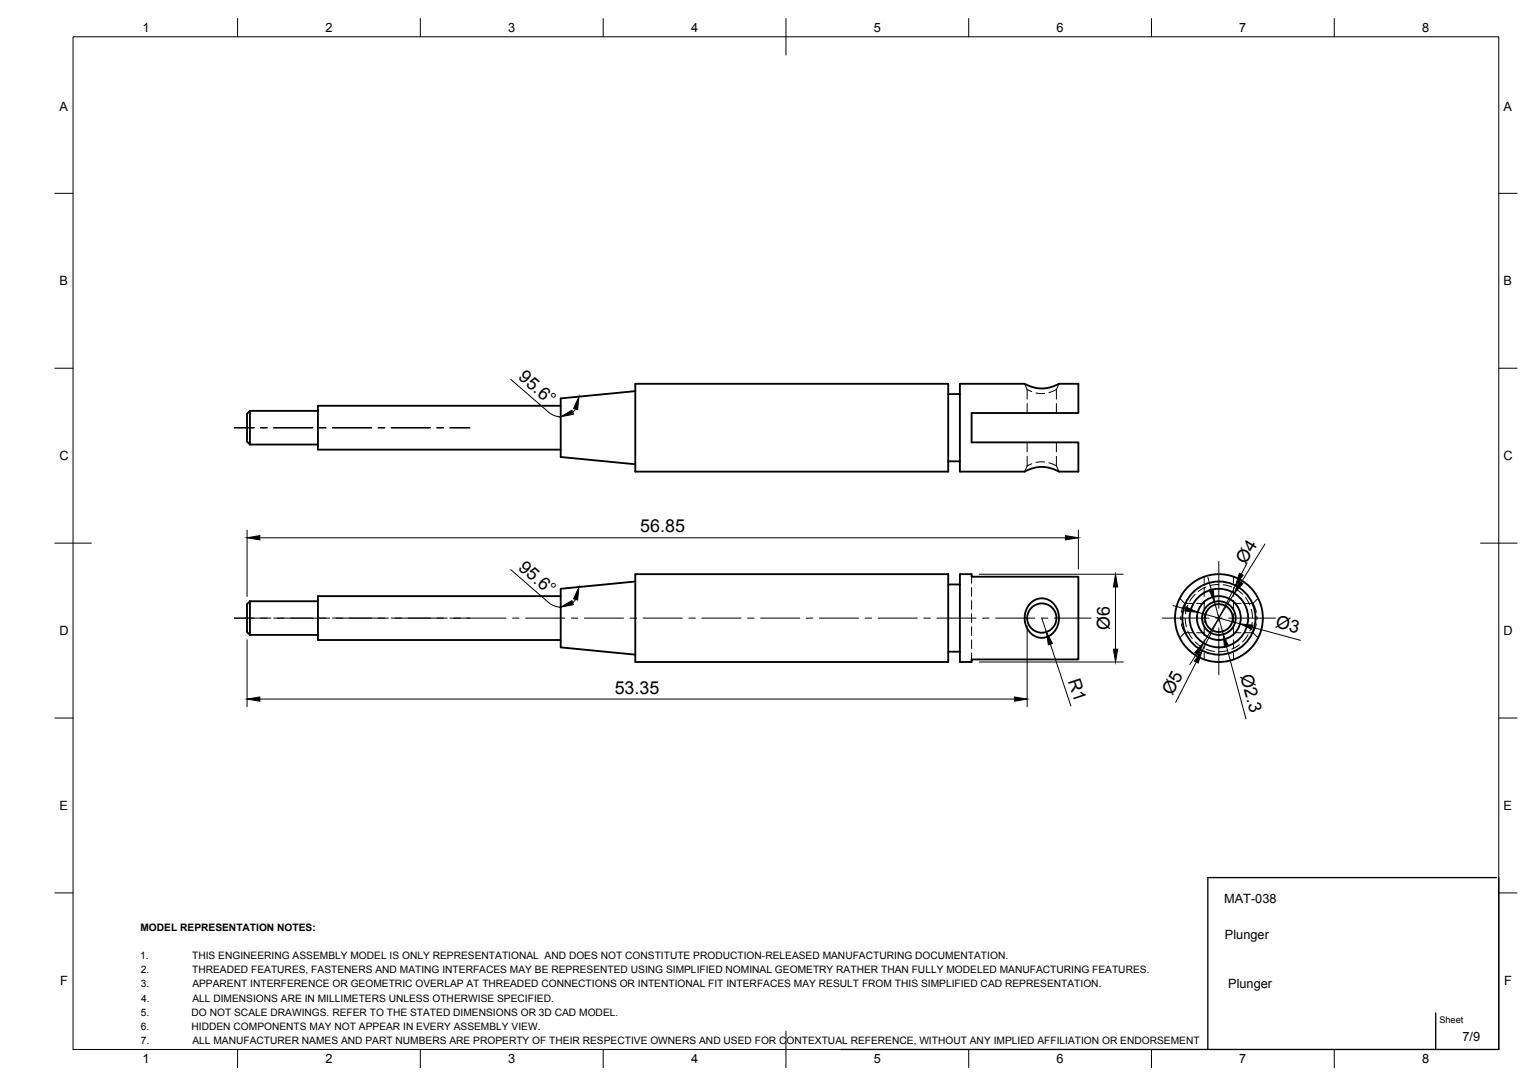
ISO-10303-21;
HEADER;
/* Generated by software containing ST-Developer
 * from STEP Tools, Inc. (www.steptools.com) 
 */

FILE_DESCRIPTION(
/* description */ ('STEP AP214'),
/* implementation_level */ '2;1');

FILE_NAME(
/* name */ 'Plunger.step',
/* time_stamp */ '2026-11-14T21:32:33-08:00',
/* author */ (''),
/* organization */ (''),
/* preprocessor_version */ 'ST-DEVELOPER v20.2',
/* originating_system */ 'Autodesk Translation Framework v15.17.0.0',
/* authorisation */ '');

FILE_SCHEMA (('AUTOMOTIVE_DESIGN { 1 0 10303 214 3 1 1 }'));
ENDSEC;

DATA;
#10=MECHANICAL_DESIGN_GEOMETRIC_PRESENTATION_REPRESENTATION('',(#181),#10551);
#135=CONICAL_SURFACE('',#3666,1.14999999999999,0.785398163397463);
#136=CONICAL_SURFACE('',#3674,1.99999999999999,0.0977269073587189);
#138=B_SPLINE_CURVE_WITH_KNOTS('',3,(#6086,#6087,#6088,#6089,#6090,#6091,
#6092,#6093,#6094,#6095,#6096,#6097,#6098,#6099,#6100,#6101,#6102,#6103,
#6104,#6105,#6106,#6107),.UNSPECIFIED.,.F.,.F.,(4,2,2,2,2,2,2,2,2,2,4),
(-0.398476386723121,-0.363413449903791,-0.328945780906488,-0.279734113540581,
-0.238759142767186,-0.202537073889496,-0.166278974820396,-0.125546922866738,
-0.0748109574930432,-0.0377065280884949,0.),.UNSPECIFIED.);
#139=B_SPLINE_CURVE_WITH_KNOTS('',3,(#6111,#6112,#6113,#6114),
 .UNSPECIFIED.,.F.,.F.,(4,4),(-0.320868204557424,-0.320859930375376),
 .UNSPECIFIED.);
#140=B_SPLINE_CURVE_WITH_KNOTS('',3,(#6116,#6117,#6118,#6119,#6120,#6121,
#6122,#6123,#6124,#6125,#6126,#6127,#6128,#6129,#6130,#6131,#6132,#6133,
#6134,#6135,#6136,#6137,#6138,#6139),.UNSPECIFIED.,.F.,.F.,(4,2,2,2,2,2,
2,2,2,2,2,4),(-0.320859930375376,-0.303821997926792,-0.286725131861031,
-0.252375001979002,-0.231369369238555,-0.194211321091721,-0.160393271457449,
-0.126524952102273,-0.0894197007003378,-0.0475320396288663,-0.0237192939459634,
-1.00000035202497E-6),.UNSPECIFIED.);
#141=B_SPLINE_CURVE_WITH_KNOTS('',3,(#6635,#6636,#6637,#6638,#6639,#6640,
#6641,#6642,#6643,#6644,#6645,#6646,#6647,#6648,#6649,#6650,#6651,#6652,
#6653,#6654,#6655,#6656),.UNSPECIFIED.,.F.,.F.,(4,2,2,2,2,2,2,2,2,2,4),
(-0.398476386717938,-0.363413449898109,-0.328945780900276,-0.279734113534564,
-0.238759142762232,-0.202537073885482,-0.166278974817291,-0.125546922864936,
-0.074810957492591,-0.0377065280884339,0.),.UNSPECIFIED.);
#142=B_SPLINE_CURVE_WITH_KNOTS('',3,(#6660,#6661,#6662,#6663),
 .UNSPECIFIED.,.F.,.F.,(4,4),(-0.320868204532271,-0.320859930350223),
 .UNSPECIFIED.);
#143=B_SPLINE_CURVE_WITH_KNOTS('',3,(#6665,#6666,#6667,#6668,#6669,#6670,
#6671,#6672,#6673,#6674,#6675,#6676,#6677,#6678,#6679,#6680,#6681,#6682,
#6683,#6684,#6685,#6686,#6687,#6688),.UNSPECIFIED.,.F.,.F.,(4,2,2,2,2,2,
2,2,2,2,2,4),(-0.320859930350223,-0.303821997902903,-0.286725131838533,
-0.252375001959359,-0.23136936922067,-0.194211321076927,-0.160393271445428,
-0.126524952093029,-0.0894197006941437,-0.0475320396261598,-0.0237192939451105,
-1.00000035191394E-6),.UNSPECIFIED.);
#144=B_SPLINE_CURVE_WITH_KNOTS('',3,(#6712,#6713,#6714,#6715,#6716,#6717,
#6718,#6719,#6720,#6721,#6722,#6723,#6724,#6725,#6726,#6727,#6728,#6729,
#6730,#6731,#6732,#6733),.UNSPECIFIED.,.F.,.F.,(4,2,2,2,2,2,2,2,2,2,4),
(-0.420674421775538,-0.382950410823496,-0.345914295714904,-0.296541537335382,
-0.257099730998724,-0.212666956872446,-0.167430581836075,-0.126839008921964,
-0.0765690827106126,-0.0387810619783508,0.),.UNSPECIFIED.);
#145=B_SPLINE_CURVE_WITH_KNOTS('',3,(#6734,#6735,#6736,#6737,#6738,#6739,
#6740,#6741,#6742,#6743,#6744,#6745,#6746,#6747,#6748,#6749,#6750,#6751,
#6752,#6753,#6754,#6755),.UNSPECIFIED.,.F.,.F.,(4,2,2,2,2,2,2,2,2,2,4),
(-0.420674421739622,-0.382950410793912,-0.345914295692047,-0.296541537321962,
-0.257099730993021,-0.212666956872502,-0.1674305818364,-0.126839008922401,
-0.0765690827112369,-0.0387810619787167,0.),.UNSPECIFIED.);
#146=B_SPLINE_CURVE_WITH_KNOTS('',3,(#6760,#6761,#6762,#6763,#6764,#6765,
#6766,#6767,#6768,#6769,#6770,#6771,#6772,#6773,#6774,#6775,#6776,#6777,
#6778,#6779,#6780,#6781),.UNSPECIFIED.,.F.,.F.,(4,2,2,2,2,2,2,2,2,2,4),
(1.00000051704647E-6,0.0346979268821443,0.0692680598480025,0.109244972085431,
0.144041383182867,0.160697846212527,0.177234449156828,0.212032576255554,
0.252099494752921,0.286510766916454,0.320844032281287),.UNSPECIFIED.);
#147=B_SPLINE_CURVE_WITH_KNOTS('',3,(#6786,#6787,#6788,#6789,#6790,#6791,
#6792,#6793,#6794,#6795,#6796,#6797,#6798,#6799,#6800,#6801,#6802,#6803,
#6804,#6805,#6806,#6807),.UNSPECIFIED.,.F.,.F.,(4,2,2,2,2,2,2,2,2,2,4),
(1.00000051707666E-6,0.0346979268820894,0.0692680598476906,0.109244972084642,
0.14404138318175,0.160697846211195,0.17723444915527,0.212032576253597,0.252099494750475,
0.286510766913486,0.3208440322786),.UNSPECIFIED.);
#155=B_SPLINE_SURFACE_WITH_KNOTS('',1,3,((#5592,#5593,#5594,#5595,#5596,
#5597,#5598,#5599,#5600,#5601,#5602,#5603,#5604,#5605,#5606,#5607,#5608,
#5609,#5610,#5611,#5612,#5613,#5614,#5615,#5616,#5617,#5618,#5619,#5620,
#5621,#5622,#5623,#5624,#5625,#5626,#5627,#5628,#5629,#5630,#5631,#5632,
#5633,#5634,#5635,#5636,#5637,#5638,#5639,#5640,#5641,#5642,#5643,#5644,
#5645,#5646,#5647,#5648,#5649,#5650,#5651,#5652,#5653,#5654,#5655,#5656,
#5657,#5658,#5659,#5660,#5661,#5662,#5663,#5664,#5665,#5666,#5667,#5668,
#5669,#5670,#5671,#5672,#5673,#5674,#5675,#5676,#5677,#5678,#5679,#5680,
#5681,#5682,#5683,#5684,#5685,#5686,#5687,#5688,#5689,#5690,#5691,#5692,
#5693,#5694,#5695,#5696,#5697,#5698,#5699,#5700,#5701,#5702,#5703,#5704,
#5705,#5706,#5707,#5708,#5709,#5710,#5711,#5712,#5713,#5714,#5715,#5716,
#5717,#5718,#5719,#5720,#5721,#5722,#5723,#5724,#5725,#5726,#5727,#5728,
#5729,#5730,#5731,#5732,#5733,#5734,#5735,#5736,#5737,#5738,#5739,#5740,
#5741,#5742,#5743,#5744,#5745,#5746,#5747,#5748,#5749,#5750,#5751,#5752,
#5753,#5754,#5755,#5756,#5757,#5758,#5759,#5760,#5761,#5762,#5763,#5764,
#5765,#5766,#5767,#5768,#5769,#5770,#5771,#5772,#5773,#5774,#5775,#5776,
#5777,#5778,#5779,#5780,#5781,#5782,#5783,#5784,#5785,#5786,#5787,#5788,
#5789,#5790,#5791,#5792,#5793,#5794,#5795,#5796,#5797,#5798,#5799,#5800,
#5801,#5802,#5803,#5804,#5805,#5806,#5807,#5808,#5809,#5810,#5811,#5812,
#5813,#5814,#5815,#5816,#5817,#5818,#5819,#5820,#5821,#5822,#5823,#5824,
#5825,#5826,#5827,#5828,#5829,#5830,#5831,#5832,#5833,#5834,#5835,#5836,
#5837),(#5838,#5839,#5840,#5841,#5842,#5843,#5844,#5845,#5846,#5847,#5848,
#5849,#5850,#5851,#5852,#5853,#5854,#5855,#5856,#5857,#5858,#5859,#5860,
#5861,#5862,#5863,#5864,#5865,#5866,#5867,#5868,#5869,#5870,#5871,#5872,
#5873,#5874,#5875,#5876,#5877,#5878,#5879,#5880,#5881,#5882,#5883,#5884,
#5885,#5886,#5887,#5888,#5889,#5890,#5891,#5892,#5893,#5894,#5895,#5896,
#5897,#5898,#5899,#5900,#5901,#5902,#5903,#5904,#5905,#5906,#5907,#5908,
#5909,#5910,#5911,#5912,#5913,#5914,#5915,#5916,#5917,#5918,#5919,#5920,
#5921,#5922,#5923,#5924,#5925,#5926,#5927,#5928,#5929,#5930,#5931,#5932,
#5933,#5934,#5935,#5936,#5937,#5938,#5939,#5940,#5941,#5942,#5943,#5944,
#5945,#5946,#5947,#5948,#5949,#5950,#5951,#5952,#5953,#5954,#5955,#5956,
#5957,#5958,#5959,#5960,#5961,#5962,#5963,#5964,#5965,#5966,#5967,#5968,
#5969,#5970,#5971,#5972,#5973,#5974,#5975,#5976,#5977,#5978,#5979,#5980,
#5981,#5982,#5983,#5984,#5985,#5986,#5987,#5988,#5989,#5990,#5991,#5992,
#5993,#5994,#5995,#5996,#5997,#5998,#5999,#6000,#6001,#6002,#6003,#6004,
#6005,#6006,#6007,#6008,#6009,#6010,#6011,#6012,#6013,#6014,#6015,#6016,
#6017,#6018,#6019,#6020,#6021,#6022,#6023,#6024,#6025,#6026,#6027,#6028,
#6029,#6030,#6031,#6032,#6033,#6034,#6035,#6036,#6037,#6038,#6039,#6040,
#6041,#6042,#6043,#6044,#6045,#6046,#6047,#6048,#6049,#6050,#6051,#6052,
#6053,#6054,#6055,#6056,#6057,#6058,#6059,#6060,#6061,#6062,#6063,#6064,
#6065,#6066,#6067,#6068,#6069,#6070,#6071,#6072,#6073,#6074,#6075,#6076,
#6077,#6078,#6079,#6080,#6081,#6082,#6083)),.UNSPECIFIED.,.F.,.T.,.F.,(2,
2),(4,2,2,2,2,2,2,2,2,2,2,2,2,2,2,2,2,2,2,2,2,2,2,2,2,2,2,2,2,2,2,2,2,2,
2,2,2,2,2,2,2,2,2,2,2,2,2,2,2,2,2,2,2,2,2,2,2,2,2,2,2,2,2,2,2,2,2,2,2,2,
2,2,2,2,2,2,2,2,2,2,2,2,2,2,2,2,2,2,2,2,2,2,2,2,2,2,2,2,2,2,2,2,2,2,2,2,
2,2,2,2,2,2,2,2,2,2,2,2,2,2,2,2,4),(-1.00016962386399E-6,1.),(0.000438425814883596,
0.00049639971234602,0.000554373609808444,0.000670321404733293,0.000728295302195718,
0.00075728225092693,0.000786269199658142,0.000844243097120567,0.000902216994582991,
0.00101816478950784,0.00107613868697026,0.00113411258443269,0.00119208648189511,
0.00125006037935754,0.00136600817428239,0.00142398207174481,0.00148195596920724,
0.00153992986666966,0.00159790376413208,0.00165587766159451,0.00171385155905693,
0.00182979935398178,0.00188777325144421,0.00191676020017542,0.00194574714890663,
0.00200372104636906,0.00206169494383148,0.00217764273875633,0.00223561663621875,
0.00229359053368118,0.0023515644311436,0.00240953832860603,0.00246751222606845,
0.00252548612353088,0.00264143391845572,0.00267042086718694,0.00269940781591815,
0.00275738171338057,0.002815355610843,0.00287332950830542,0.00293130340576785,
0.00298927730323027,0.0030472512006927,0.00310522509815512,0.00316319899561754,
0.00322117289307997,0.00333712068800482,0.00339509458546724,0.00342408153419845,
0.00345306848292967,0.00351104238039209,0.00356901627785452,0.00368496407277936,
0.00380091186770421,0.00385888576516664,0.00391685966262906,0.00397483356009149,
0.00403280745755391,0.00414875525247876,0.00420672914994119,0.00426470304740361,
0.00432267694486603,0.00438065084232846,0.00443862473979088,0.00449659863725331,
0.00461254643217816,0.00467052032964058,0.00469950727837179,0.00472849422710301,
0.00478646812456543,0.00484444202202785,0.0049603898169527,0.00501836371441513,
0.00507633761187755,0.00510532456060876,0.00513431150933998,0.0051922854068024,
0.00530823320172725,0.00536620709918968,0.0054241809966521,0.00548215489411452,
0.00551114184284574,0.00554012879157695,0.0056560765865018,0.00577202438142665,
0.00582999827888907,0.00588797217635149,0.00591695912508271,0.00594594607381392,
0.00600391997127634,0.00611986776620119,0.00617784166366362,0.00623581556112604,
0.00626480250985725,0.00629378945858847,0.00635176335605089,0.00640973725351331,
0.00646771115097574,0.00658365894590059,0.0066126458946318,0.00664163284336301,
0.00669960674082544,0.00675758063828786,0.00681555453575028,0.00687352843321271,
0.00693150233067513,0.00698947622813756,0.00701846317686877,0.00704745012559998,
0.00716339792052483,0.00727934571544968,0.0073373196129121,0.00739529351037453,
0.00742428045910574,0.00745326740783695,0.00751124130529938,0.0075692152027618,
0.00762718910022423,0.00768516299768665,0.00774313689514908,0.0078011107926115,
0.00783009774134271,0.00785908469007393),.UNSPECIFIED.);
#156=B_SPLINE_SURFACE_WITH_KNOTS('',1,3,((#6141,#6142,#6143,#6144,#6145,
#6146,#6147,#6148,#6149,#6150,#6151,#6152,#6153,#6154,#6155,#6156,#6157,
#6158,#6159,#6160,#6161,#6162,#6163,#6164,#6165,#6166,#6167,#6168,#6169,
#6170,#6171,#6172,#6173,#6174,#6175,#6176,#6177,#6178,#6179,#6180,#6181,
#6182,#6183,#6184,#6185,#6186,#6187,#6188,#6189,#6190,#6191,#6192,#6193,
#6194,#6195,#6196,#6197,#6198,#6199,#6200,#6201,#6202,#6203,#6204,#6205,
#6206,#6207,#6208,#6209,#6210,#6211,#6212,#6213,#6214,#6215,#6216,#6217,
#6218,#6219,#6220,#6221,#6222,#6223,#6224,#6225,#6226,#6227,#6228,#6229,
#6230,#6231,#6232,#6233,#6234,#6235,#6236,#6237,#6238,#6239,#6240,#6241,
#6242,#6243,#6244,#6245,#6246,#6247,#6248,#6249,#6250,#6251,#6252,#6253,
#6254,#6255,#6256,#6257,#6258,#6259,#6260,#6261,#6262,#6263,#6264,#6265,
#6266,#6267,#6268,#6269,#6270,#6271,#6272,#6273,#6274,#6275,#6276,#6277,
#6278,#6279,#6280,#6281,#6282,#6283,#6284,#6285,#6286,#6287,#6288,#6289,
#6290,#6291,#6292,#6293,#6294,#6295,#6296,#6297,#6298,#6299,#6300,#6301,
#6302,#6303,#6304,#6305,#6306,#6307,#6308,#6309,#6310,#6311,#6312,#6313,
#6314,#6315,#6316,#6317,#6318,#6319,#6320,#6321,#6322,#6323,#6324,#6325,
#6326,#6327,#6328,#6329,#6330,#6331,#6332,#6333,#6334,#6335,#6336,#6337,
#6338,#6339,#6340,#6341,#6342,#6343,#6344,#6345,#6346,#6347,#6348,#6349,
#6350,#6351,#6352,#6353,#6354,#6355,#6356,#6357,#6358,#6359,#6360,#6361,
#6362,#6363,#6364,#6365,#6366,#6367,#6368,#6369,#6370,#6371,#6372,#6373,
#6374,#6375,#6376,#6377,#6378,#6379,#6380,#6381,#6382,#6383,#6384,#6385,
#6386),(#6387,#6388,#6389,#6390,#6391,#6392,#6393,#6394,#6395,#6396,#6397,
#6398,#6399,#6400,#6401,#6402,#6403,#6404,#6405,#6406,#6407,#6408,#6409,
#6410,#6411,#6412,#6413,#6414,#6415,#6416,#6417,#6418,#6419,#6420,#6421,
#6422,#6423,#6424,#6425,#6426,#6427,#6428,#6429,#6430,#6431,#6432,#6433,
#6434,#6435,#6436,#6437,#6438,#6439,#6440,#6441,#6442,#6443,#6444,#6445,
#6446,#6447,#6448,#6449,#6450,#6451,#6452,#6453,#6454,#6455,#6456,#6457,
#6458,#6459,#6460,#6461,#6462,#6463,#6464,#6465,#6466,#6467,#6468,#6469,
#6470,#6471,#6472,#6473,#6474,#6475,#6476,#6477,#6478,#6479,#6480,#6481,
#6482,#6483,#6484,#6485,#6486,#6487,#6488,#6489,#6490,#6491,#6492,#6493,
#6494,#6495,#6496,#6497,#6498,#6499,#6500,#6501,#6502,#6503,#6504,#6505,
#6506,#6507,#6508,#6509,#6510,#6511,#6512,#6513,#6514,#6515,#6516,#6517,
#6518,#6519,#6520,#6521,#6522,#6523,#6524,#6525,#6526,#6527,#6528,#6529,
#6530,#6531,#6532,#6533,#6534,#6535,#6536,#6537,#6538,#6539,#6540,#6541,
#6542,#6543,#6544,#6545,#6546,#6547,#6548,#6549,#6550,#6551,#6552,#6553,
#6554,#6555,#6556,#6557,#6558,#6559,#6560,#6561,#6562,#6563,#6564,#6565,
#6566,#6567,#6568,#6569,#6570,#6571,#6572,#6573,#6574,#6575,#6576,#6577,
#6578,#6579,#6580,#6581,#6582,#6583,#6584,#6585,#6586,#6587,#6588,#6589,
#6590,#6591,#6592,#6593,#6594,#6595,#6596,#6597,#6598,#6599,#6600,#6601,
#6602,#6603,#6604,#6605,#6606,#6607,#6608,#6609,#6610,#6611,#6612,#6613,
#6614,#6615,#6616,#6617,#6618,#6619,#6620,#6621,#6622,#6623,#6624,#6625,
#6626,#6627,#6628,#6629,#6630,#6631,#6632)),.UNSPECIFIED.,.F.,.T.,.F.,(2,
2),(4,2,2,2,2,2,2,2,2,2,2,2,2,2,2,2,2,2,2,2,2,2,2,2,2,2,2,2,2,2,2,2,2,2,
2,2,2,2,2,2,2,2,2,2,2,2,2,2,2,2,2,2,2,2,2,2,2,2,2,2,2,2,2,2,2,2,2,2,2,2,
2,2,2,2,2,2,2,2,2,2,2,2,2,2,2,2,2,2,2,2,2,2,2,2,2,2,2,2,2,2,2,2,2,2,2,2,
2,2,2,2,2,2,2,2,2,2,2,2,2,2,2,2,4),(-1.00016962714665E-6,1.),(0.000438425814883592,
0.000496399712346016,0.000554373609808441,0.000670321404733289,0.000728295302195713,
0.000757282250926925,0.000786269199658137,0.000844243097120562,0.000902216994582986,
0.00101816478950783,0.00107613868697026,0.00113411258443268,0.00119208648189511,
0.00125006037935753,0.00136600817428238,0.0014239820717448,0.00148195596920723,
0.00153992986666965,0.00159790376413208,0.0016558776615945,0.00171385155905693,
0.00182979935398177,0.0018877732514442,0.00191676020017541,0.00194574714890662,
0.00200372104636905,0.00206169494383147,0.00217764273875632,0.00223561663621874,
0.00229359053368117,0.00235156443114359,0.00240953832860602,0.00246751222606844,
0.00252548612353086,0.00264143391845571,0.00267042086718692,0.00269940781591814,
0.00275738171338056,0.00281535561084298,0.00287332950830541,0.00293130340576783,
0.00298927730323026,0.00304725120069268,0.00310522509815511,0.00316319899561753,
0.00322117289307996,0.0033371206880048,0.00339509458546723,0.00342408153419844,
0.00345306848292965,0.00351104238039208,0.0035690162778545,0.00368496407277935,
0.0038009118677042,0.00385888576516662,0.00391685966262905,0.00397483356009147,
0.00403280745755389,0.00414875525247874,0.00420672914994117,0.00426470304740359,
0.00432267694486602,0.00438065084232844,0.00443862473979086,0.00449659863725329,
0.00461254643217814,0.00467052032964056,0.00469950727837177,0.00472849422710298,
0.00478646812456541,0.00484444202202783,0.00496038981695268,0.00501836371441511,
0.00507633761187753,0.00510532456060874,0.00513431150933995,0.00519228540680238,
0.00530823320172723,0.00536620709918965,0.00542418099665208,0.0054821548941145,
0.00551114184284571,0.00554012879157692,0.00565607658650177,0.00577202438142662,
0.00582999827888904,0.00588797217635147,0.00591695912508268,0.00594594607381389,
0.00600391997127632,0.00611986776620117,0.00617784166366359,0.00623581556112602,
0.00626480250985723,0.00629378945858844,0.00635176335605086,0.00640973725351329,
0.00646771115097571,0.00658365894590056,0.00661264589463177,0.00664163284336298,
0.00669960674082541,0.00675758063828783,0.00681555453575026,0.00687352843321268,
0.00693150233067511,0.00698947622813753,0.00701846317686874,0.00704745012559995,
0.0071633979205248,0.00727934571544965,0.00733731961291207,0.0073952935103745,
0.00742428045910571,0.00745326740783692,0.00751124130529935,0.00756921520276177,
0.0076271891002242,0.00768516299768662,0.00774313689514904,0.00780111079261147,
0.00783009774134268,0.00785908469007389),.UNSPECIFIED.);
#157=B_SPLINE_SURFACE_WITH_KNOTS('',1,3,((#6848,#6849,#6850,#6851,#6852,
#6853,#6854,#6855,#6856,#6857,#6858,#6859,#6860,#6861,#6862,#6863,#6864,
#6865,#6866,#6867,#6868,#6869,#6870,#6871,#6872,#6873,#6874,#6875,#6876,
#6877,#6878,#6879,#6880,#6881,#6882,#6883,#6884,#6885,#6886,#6887,#6888,
#6889,#6890,#6891,#6892,#6893,#6894,#6895,#6896,#6897,#6898,#6899,#6900,
#6901,#6902,#6903,#6904,#6905,#6906,#6907,#6908,#6909,#6910,#6911,#6912,
#6913,#6914,#6915,#6916,#6917,#6918,#6919,#6920,#6921,#6922,#6923,#6924,
#6925,#6926,#6927,#6928,#6929,#6930,#6931,#6932,#6933,#6934,#6935,#6936,
#6937,#6938,#6939,#6940,#6941,#6942,#6943,#6944,#6945,#6946,#6947,#6948,
#6949,#6950,#6951,#6952,#6953,#6954,#6955,#6956,#6957,#6958,#6959,#6960,
#6961,#6962,#6963,#6964,#6965,#6966,#6967,#6968,#6969,#6970,#6971,#6972,
#6973,#6974,#6975,#6976,#6977,#6978,#6979,#6980,#6981,#6982,#6983,#6984,
#6985,#6986,#6987,#6988,#6989,#6990,#6991,#6992,#6993,#6994,#6995,#6996,
#6997,#6998,#6999,#7000,#7001,#7002,#7003,#7004,#7005,#7006,#7007,#7008,
#7009,#7010,#7011,#7012,#7013,#7014,#7015,#7016,#7017,#7018,#7019,#7020,
#7021,#7022,#7023,#7024,#7025,#7026,#7027,#7028,#7029,#7030,#7031,#7032,
#7033,#7034,#7035,#7036,#7037,#7038,#7039,#7040,#7041,#7042,#7043,#7044,
#7045,#7046,#7047,#7048,#7049,#7050,#7051,#7052,#7053,#7054,#7055,#7056,
#7057,#7058,#7059,#7060,#7061,#7062,#7063,#7064,#7065,#7066,#7067,#7068,
#7069,#7070,#7071,#7072,#7073,#7074,#7075,#7076,#7077,#7078,#7079,#7080,
#7081,#7082,#7083,#7084,#7085,#7086,#7087,#7088,#7089,#7090,#7091,#7092,
#7093),(#7094,#7095,#7096,#7097,#7098,#7099,#7100,#7101,#7102,#7103,#7104,
#7105,#7106,#7107,#7108,#7109,#7110,#7111,#7112,#7113,#7114,#7115,#7116,
#7117,#7118,#7119,#7120,#7121,#7122,#7123,#7124,#7125,#7126,#7127,#7128,
#7129,#7130,#7131,#7132,#7133,#7134,#7135,#7136,#7137,#7138,#7139,#7140,
#7141,#7142,#7143,#7144,#7145,#7146,#7147,#7148,#7149,#7150,#7151,#7152,
#7153,#7154,#7155,#7156,#7157,#7158,#7159,#7160,#7161,#7162,#7163,#7164,
#7165,#7166,#7167,#7168,#7169,#7170,#7171,#7172,#7173,#7174,#7175,#7176,
#7177,#7178,#7179,#7180,#7181,#7182,#7183,#7184,#7185,#7186,#7187,#7188,
#7189,#7190,#7191,#7192,#7193,#7194,#7195,#7196,#7197,#7198,#7199,#7200,
#7201,#7202,#7203,#7204,#7205,#7206,#7207,#7208,#7209,#7210,#7211,#7212,
#7213,#7214,#7215,#7216,#7217,#7218,#7219,#7220,#7221,#7222,#7223,#7224,
#7225,#7226,#7227,#7228,#7229,#7230,#7231,#7232,#7233,#7234,#7235,#7236,
#7237,#7238,#7239,#7240,#7241,#7242,#7243,#7244,#7245,#7246,#7247,#7248,
#7249,#7250,#7251,#7252,#7253,#7254,#7255,#7256,#7257,#7258,#7259,#7260,
#7261,#7262,#7263,#7264,#7265,#7266,#7267,#7268,#7269,#7270,#7271,#7272,
#7273,#7274,#7275,#7276,#7277,#7278,#7279,#7280,#7281,#7282,#7283,#7284,
#7285,#7286,#7287,#7288,#7289,#7290,#7291,#7292,#7293,#7294,#7295,#7296,
#7297,#7298,#7299,#7300,#7301,#7302,#7303,#7304,#7305,#7306,#7307,#7308,
#7309,#7310,#7311,#7312,#7313,#7314,#7315,#7316,#7317,#7318,#7319,#7320,
#7321,#7322,#7323,#7324,#7325,#7326,#7327,#7328,#7329,#7330,#7331,#7332,
#7333,#7334,#7335,#7336,#7337,#7338,#7339)),.UNSPECIFIED.,.F.,.T.,.F.,(2,
2),(4,2,2,2,2,2,2,2,2,2,2,2,2,2,2,2,2,2,2,2,2,2,2,2,2,2,2,2,2,2,2,2,2,2,
2,2,2,2,2,2,2,2,2,2,2,2,2,2,2,2,2,2,2,2,2,2,2,2,2,2,2,2,2,2,2,2,2,2,2,2,
2,2,2,2,2,2,2,2,2,2,2,2,2,2,2,2,2,2,2,2,2,2,2,2,2,2,2,2,2,2,2,2,2,2,2,2,
2,2,2,2,2,2,2,2,2,2,2,2,2,2,2,2,4),(-3.16760819181413E-6,1.00000897992091),
(0.000438425814883592,0.000496399712346016,0.000554373609808441,0.000670321404733289,
0.000728295302195713,0.000757282250926925,0.000786269199658137,0.000844243097120562,
0.000902216994582986,0.00101816478950783,0.00107613868697026,0.00113411258443268,
0.00119208648189511,0.00125006037935753,0.00136600817428238,0.0014239820717448,
0.00148195596920723,0.00153992986666965,0.00159790376413208,0.0016558776615945,
0.00171385155905693,0.00182979935398177,0.0018877732514442,0.00191676020017541,
0.00194574714890662,0.00200372104636905,0.00206169494383147,0.00217764273875632,
0.00223561663621874,0.00229359053368117,0.00235156443114359,0.00240953832860602,
0.00246751222606844,0.00252548612353086,0.00264143391845571,0.00267042086718692,
0.00269940781591814,0.00275738171338056,0.00281535561084298,0.00287332950830541,
0.00293130340576783,0.00298927730323026,0.00304725120069268,0.00310522509815511,
0.00316319899561753,0.00322117289307996,0.0033371206880048,0.00339509458546723,
0.00342408153419844,0.00345306848292965,0.00351104238039208,0.0035690162778545,
0.00368496407277935,0.0038009118677042,0.00385888576516662,0.00391685966262905,
0.00397483356009147,0.00403280745755389,0.00414875525247874,0.00420672914994117,
0.00426470304740359,0.00432267694486602,0.00438065084232844,0.00443862473979086,
0.00449659863725329,0.00461254643217814,0.00467052032964056,0.00469950727837177,
0.00472849422710298,0.00478646812456541,0.00484444202202783,0.00496038981695268,
0.00501836371441511,0.00507633761187753,0.00510532456060874,0.00513431150933995,
0.00519228540680238,0.00530823320172723,0.00536620709918965,0.00542418099665208,
0.0054821548941145,0.00551114184284571,0.00554012879157692,0.00565607658650177,
0.00577202438142662,0.00582999827888904,0.00588797217635147,0.00591695912508268,
0.00594594607381389,0.00600391997127632,0.00611986776620117,0.00617784166366359,
0.00623581556112602,0.00626480250985723,0.00629378945858844,0.00635176335605086,
0.00640973725351329,0.00646771115097571,0.00658365894590056,0.00661264589463177,
0.00664163284336298,0.00669960674082541,0.00675758063828783,0.00681555453575026,
0.00687352843321268,0.00693150233067511,0.00698947622813753,0.00701846317686874,
0.00704745012559995,0.0071633979205248,0.00727934571544965,0.00733731961291207,
0.0073952935103745,0.00742428045910571,0.00745326740783692,0.00751124130529935,
0.00756921520276177,0.0076271891002242,0.00768516299768662,0.00774313689514904,
0.00780111079261147,0.00783009774134268,0.00785908469007389),
 .UNSPECIFIED.);
#158=B_SPLINE_SURFACE_WITH_KNOTS('',1,3,((#7340,#7341,#7342,#7343,#7344,
#7345,#7346,#7347,#7348,#7349,#7350,#7351,#7352,#7353,#7354,#7355,#7356,
#7357,#7358,#7359,#7360,#7361,#7362,#7363,#7364,#7365,#7366,#7367,#7368,
#7369,#7370,#7371,#7372,#7373,#7374,#7375,#7376,#7377,#7378,#7379,#7380,
#7381,#7382,#7383,#7384,#7385,#7386,#7387,#7388,#7389,#7390,#7391,#7392,
#7393,#7394,#7395,#7396,#7397,#7398,#7399,#7400,#7401,#7402,#7403,#7404,
#7405,#7406,#7407,#7408,#7409,#7410,#7411,#7412,#7413,#7414,#7415,#7416,
#7417,#7418,#7419,#7420,#7421,#7422,#7423,#7424,#7425,#7426,#7427,#7428,
#7429,#7430,#7431,#7432,#7433,#7434,#7435,#7436,#7437,#7438,#7439,#7440,
#7441,#7442,#7443,#7444,#7445,#7446,#7447,#7448,#7449,#7450,#7451,#7452,
#7453,#7454,#7455,#7456,#7457,#7458,#7459,#7460,#7461,#7462,#7463,#7464,
#7465,#7466,#7467,#7468,#7469,#7470,#7471,#7472,#7473,#7474,#7475,#7476,
#7477,#7478,#7479,#7480,#7481,#7482,#7483,#7484,#7485,#7486,#7487,#7488,
#7489,#7490,#7491,#7492,#7493,#7494,#7495,#7496,#7497,#7498,#7499,#7500,
#7501,#7502,#7503,#7504,#7505,#7506,#7507,#7508,#7509,#7510,#7511,#7512,
#7513,#7514,#7515,#7516,#7517,#7518,#7519,#7520,#7521,#7522,#7523,#7524,
#7525,#7526,#7527,#7528,#7529,#7530,#7531,#7532,#7533,#7534,#7535,#7536,
#7537,#7538,#7539,#7540,#7541,#7542,#7543,#7544,#7545,#7546,#7547,#7548,
#7549,#7550,#7551,#7552,#7553,#7554,#7555,#7556,#7557,#7558,#7559,#7560,
#7561,#7562,#7563,#7564,#7565,#7566,#7567,#7568,#7569,#7570,#7571,#7572,
#7573,#7574,#7575,#7576,#7577,#7578,#7579,#7580,#7581,#7582,#7583,#7584,
#7585),(#7586,#7587,#7588,#7589,#7590,#7591,#7592,#7593,#7594,#7595,#7596,
#7597,#7598,#7599,#7600,#7601,#7602,#7603,#7604,#7605,#7606,#7607,#7608,
#7609,#7610,#7611,#7612,#7613,#7614,#7615,#7616,#7617,#7618,#7619,#7620,
#7621,#7622,#7623,#7624,#7625,#7626,#7627,#7628,#7629,#7630,#7631,#7632,
#7633,#7634,#7635,#7636,#7637,#7638,#7639,#7640,#7641,#7642,#7643,#7644,
#7645,#7646,#7647,#7648,#7649,#7650,#7651,#7652,#7653,#7654,#7655,#7656,
#7657,#7658,#7659,#7660,#7661,#7662,#7663,#7664,#7665,#7666,#7667,#7668,
#7669,#7670,#7671,#7672,#7673,#7674,#7675,#7676,#7677,#7678,#7679,#7680,
#7681,#7682,#7683,#7684,#7685,#7686,#7687,#7688,#7689,#7690,#7691,#7692,
#7693,#7694,#7695,#7696,#7697,#7698,#7699,#7700,#7701,#7702,#7703,#7704,
#7705,#7706,#7707,#7708,#7709,#7710,#7711,#7712,#7713,#7714,#7715,#7716,
#7717,#7718,#7719,#7720,#7721,#7722,#7723,#7724,#7725,#7726,#7727,#7728,
#7729,#7730,#7731,#7732,#7733,#7734,#7735,#7736,#7737,#7738,#7739,#7740,
#7741,#7742,#7743,#7744,#7745,#7746,#7747,#7748,#7749,#7750,#7751,#7752,
#7753,#7754,#7755,#7756,#7757,#7758,#7759,#7760,#7761,#7762,#7763,#7764,
#7765,#7766,#7767,#7768,#7769,#7770,#7771,#7772,#7773,#7774,#7775,#7776,
#7777,#7778,#7779,#7780,#7781,#7782,#7783,#7784,#7785,#7786,#7787,#7788,
#7789,#7790,#7791,#7792,#7793,#7794,#7795,#7796,#7797,#7798,#7799,#7800,
#7801,#7802,#7803,#7804,#7805,#7806,#7807,#7808,#7809,#7810,#7811,#7812,
#7813,#7814,#7815,#7816,#7817,#7818,#7819,#7820,#7821,#7822,#7823,#7824,
#7825,#7826,#7827,#7828,#7829,#7830,#7831)),.UNSPECIFIED.,.F.,.T.,.F.,(2,
2),(4,2,2,2,2,2,2,2,2,2,2,2,2,2,2,2,2,2,2,2,2,2,2,2,2,2,2,2,2,2,2,2,2,2,
2,2,2,2,2,2,2,2,2,2,2,2,2,2,2,2,2,2,2,2,2,2,2,2,2,2,2,2,2,2,2,2,2,2,2,2,
2,2,2,2,2,2,2,2,2,2,2,2,2,2,2,2,2,2,2,2,2,2,2,2,2,2,2,2,2,2,2,2,2,2,2,2,
2,2,2,2,2,2,2,2,2,2,2,2,2,2,2,2,4),(-3.16760819184598E-6,1.00000897992087),
(0.000438425814883596,0.00049639971234602,0.000554373609808444,0.000670321404733293,
0.000728295302195718,0.00075728225092693,0.000786269199658142,0.000844243097120567,
0.000902216994582991,0.00101816478950784,0.00107613868697026,0.00113411258443269,
0.00119208648189511,0.00125006037935754,0.00136600817428239,0.00142398207174481,
0.00148195596920724,0.00153992986666966,0.00159790376413208,0.00165587766159451,
0.00171385155905693,0.00182979935398178,0.00188777325144421,0.00191676020017542,
0.00194574714890663,0.00200372104636906,0.00206169494383148,0.00217764273875633,
0.00223561663621875,0.00229359053368118,0.0023515644311436,0.00240953832860603,
0.00246751222606845,0.00252548612353088,0.00264143391845572,0.00267042086718694,
0.00269940781591815,0.00275738171338057,0.002815355610843,0.00287332950830542,
0.00293130340576785,0.00298927730323027,0.0030472512006927,0.00310522509815512,
0.00316319899561754,0.00322117289307997,0.00333712068800482,0.00339509458546724,
0.00342408153419845,0.00345306848292967,0.00351104238039209,0.00356901627785452,
0.00368496407277936,0.00380091186770421,0.00385888576516664,0.00391685966262906,
0.00397483356009149,0.00403280745755391,0.00414875525247876,0.00420672914994119,
0.00426470304740361,0.00432267694486603,0.00438065084232846,0.00443862473979088,
0.00449659863725331,0.00461254643217816,0.00467052032964058,0.00469950727837179,
0.00472849422710301,0.00478646812456543,0.00484444202202785,0.0049603898169527,
0.00501836371441513,0.00507633761187755,0.00510532456060876,0.00513431150933998,
0.0051922854068024,0.00530823320172725,0.00536620709918968,0.0054241809966521,
0.00548215489411452,0.00551114184284574,0.00554012879157695,0.0056560765865018,
0.00577202438142665,0.00582999827888907,0.00588797217635149,0.00591695912508271,
0.00594594607381392,0.00600391997127634,0.00611986776620119,0.00617784166366362,
0.00623581556112604,0.00626480250985725,0.00629378945858847,0.00635176335605089,
0.00640973725351331,0.00646771115097574,0.00658365894590059,0.0066126458946318,
0.00664163284336301,0.00669960674082544,0.00675758063828786,0.00681555453575028,
0.00687352843321271,0.00693150233067513,0.00698947622813756,0.00701846317686877,
0.00704745012559998,0.00716339792052483,0.00727934571544968,0.0073373196129121,
0.00739529351037453,0.00742428045910574,0.00745326740783695,0.00751124130529938,
0.0075692152027618,0.00762718910022423,0.00768516299768665,0.00774313689514908,
0.0078011107926115,0.00783009774134271,0.00785908469007393),
 .UNSPECIFIED.);
#163=SHAPE_REPRESENTATION_RELATIONSHIP('SRR','None',#10590,#172);
#172=ADVANCED_BREP_SHAPE_REPRESENTATION('',(#191),#10546);
#181=STYLED_ITEM('',(#10643),#191);
#191=MANIFOLD_SOLID_BREP('Body1',#3430);
#212=FACE_BOUND('',#600,.T.);
#213=FACE_BOUND('',#601,.T.);
#214=FACE_BOUND('',#611,.T.);
#215=FACE_BOUND('',#613,.T.);
#216=FACE_BOUND('',#615,.T.);
#217=FACE_BOUND('',#618,.T.);
#218=FACE_BOUND('',#620,.T.);
#219=FACE_BOUND('',#625,.T.);
#220=FACE_BOUND('',#628,.T.);
#271=PLANE('',#3680);
#272=PLANE('',#3681);
#273=PLANE('',#3682);
#274=PLANE('',#3683);
#275=PLANE('',#3684);
#276=PLANE('',#3685);
#277=PLANE('',#3686);
#278=PLANE('',#3687);
#279=PLANE('',#3688);
#280=PLANE('',#3689);
#281=PLANE('',#3690);
#362=FACE_OUTER_BOUND('',#597,.T.);
#363=FACE_OUTER_BOUND('',#598,.T.);
#364=FACE_OUTER_BOUND('',#599,.T.);
#365=FACE_OUTER_BOUND('',#602,.T.);
#366=FACE_OUTER_BOUND('',#603,.T.);
#367=FACE_OUTER_BOUND('',#604,.T.);
#368=FACE_OUTER_BOUND('',#605,.T.);
#369=FACE_OUTER_BOUND('',#606,.T.);
#370=FACE_OUTER_BOUND('',#607,.T.);
#371=FACE_OUTER_BOUND('',#608,.T.);
#372=FACE_OUTER_BOUND('',#609,.T.);
#373=FACE_OUTER_BOUND('',#610,.T.);
#374=FACE_OUTER_BOUND('',#612,.T.);
#375=FACE_OUTER_BOUND('',#614,.T.);
#376=FACE_OUTER_BOUND('',#616,.T.);
#377=FACE_OUTER_BOUND('',#617,.T.);
#378=FACE_OUTER_BOUND('',#619,.T.);
#379=FACE_OUTER_BOUND('',#621,.T.);
#380=FACE_OUTER_BOUND('',#622,.T.);
#381=FACE_OUTER_BOUND('',#623,.T.);
#382=FACE_OUTER_BOUND('',#624,.T.);
#383=FACE_OUTER_BOUND('',#626,.T.);
#384=FACE_OUTER_BOUND('',#627,.T.);
#385=FACE_OUTER_BOUND('',#629,.T.);
#597=EDGE_LOOP('',(#2530,#2531,#2532,#2533,#2534));
#598=EDGE_LOOP('',(#2535,#2536,#2537,#2538,#2539));
#599=EDGE_LOOP('',(#2540,#2541,#2542,#2543,#2544,#2545,#2546,#2547,#2548,
#2549,#2550,#2551));
#600=EDGE_LOOP('',(#2552,#2553));
#601=EDGE_LOOP('',(#2554,#2555));
#602=EDGE_LOOP('',(#2556,#2557,#2558,#2559,#2560,#2561));
#603=EDGE_LOOP('',(#2562,#2563,#2564,#2565,#2566,#2567));
#604=EDGE_LOOP('',(#2568,#2569,#2570,#2571));
#605=EDGE_LOOP('',(#2572,#2573,#2574,#2575));
#606=EDGE_LOOP('',(#2576,#2577,#2578,#2579));
#607=EDGE_LOOP('',(#2580,#2581,#2582,#2583));
#608=EDGE_LOOP('',(#2584,#2585,#2586,#2587));
#609=EDGE_LOOP('',(#2588,#2589,#2590,#2591));
#610=EDGE_LOOP('',(#2592));
#611=EDGE_LOOP('',(#2593));
#612=EDGE_LOOP('',(#2594));
#613=EDGE_LOOP('',(#2595));
#614=EDGE_LOOP('',(#2596));
#615=EDGE_LOOP('',(#2597));
#616=EDGE_LOOP('',(#2598));
#617=EDGE_LOOP('',(#2599));
#618=EDGE_LOOP('',(#2600));
#619=EDGE_LOOP('',(#2601));
#620=EDGE_LOOP('',(#2602));
#621=EDGE_LOOP('',(#2603,#2604,#2605,#2606));
#622=EDGE_LOOP('',(#2607,#2608,#2609,#2610));
#623=EDGE_LOOP('',(#2611,#2612));
#624=EDGE_LOOP('',(#2613,#2614,#2615,#2616));
#625=EDGE_LOOP('',(#2617));
#626=EDGE_LOOP('',(#2618,#2619,#2620,#2621,#2622));
#627=EDGE_LOOP('',(#2623,#2624,#2625,#2626));
#628=EDGE_LOOP('',(#2627));
#629=EDGE_LOOP('',(#2628,#2629));
#890=LINE('',#6109,#1087);
#891=LINE('',#6140,#1088);
#892=LINE('',#6658,#1089);
#893=LINE('',#6689,#1090);
#894=LINE('',#6695,#1091);
#895=LINE('',#6699,#1092);
#896=LINE('',#6703,#1093);
#897=LINE('',#6708,#1094);
#898=LINE('',#6711,#1095);
#899=LINE('',#6758,#1096);
#900=LINE('',#6785,#1097);
#901=LINE('',#6812,#1098);
#902=LINE('',#6818,#1099);
#903=LINE('',#6823,#1100);
#904=LINE('',#6828,#1101);
#905=LINE('',#6834,#1102);
#906=LINE('',#6840,#1103);
#907=LINE('',#7833,#1104);
#908=LINE('',#7835,#1105);
#909=LINE('',#7837,#1106);
#910=LINE('',#7839,#1107);
#1087=VECTOR('',#4397,10.);
#1088=VECTOR('',#4398,10.);
#1089=VECTOR('',#4399,10.);
#1090=VECTOR('',#4400,10.);
#1091=VECTOR('',#4405,1000.);
#1092=VECTOR('',#4408,1000.);
#1093=VECTOR('',#4411,3.);
#1094=VECTOR('',#4416,1000.);
#1095=VECTOR('',#4419,1000.);
#1096=VECTOR('',#4422,1.);
#1097=VECTOR('',#4429,1.);
#1098=VECTOR('',#4434,2.3);
#1099=VECTOR('',#4441,1.14999999999999);
#1100=VECTOR('',#4448,1.14999999999999);
#1101=VECTOR('',#4453,1.49999999999999);
#1102=VECTOR('',#4460,1.99999999999999);
#1103=VECTOR('',#4467,3.);
#1104=VECTOR('',#4484,1000.);
#1105=VECTOR('',#4487,1000.);
#1106=VECTOR('',#4490,1000.);
#1107=VECTOR('',#4493,1000.);
#1197=CIRCLE('',#3653,3.);
#1198=CIRCLE('',#3654,3.);
#1199=CIRCLE('',#3655,3.);
#1200=CIRCLE('',#3656,3.);
#1201=CIRCLE('',#3657,3.);
#1202=CIRCLE('',#3658,3.);
#1203=CIRCLE('',#3660,1.);
#1204=CIRCLE('',#3662,1.);
#1205=CIRCLE('',#3664,2.3);
#1206=CIRCLE('',#3665,2.3);
#1207=CIRCLE('',#3667,1.14999999999999);
#1208=CIRCLE('',#3668,0.949999999999971);
#1209=CIRCLE('',#3670,1.14999999999999);
#1210=CIRCLE('',#3672,1.49999999999999);
#1211=CIRCLE('',#3673,1.49999999999999);
#1212=CIRCLE('',#3675,2.49999999999999);
#1213=CIRCLE('',#3676,1.99999999999999);
#1214=CIRCLE('',#3678,3.);
#1215=CIRCLE('',#3679,2.99999999999999);
#1535=VERTEX_POINT('',#6084);
#1536=VERTEX_POINT('',#6085);
#1537=VERTEX_POINT('',#6108);
#1538=VERTEX_POINT('',#6110);
#1539=VERTEX_POINT('',#6115);
#1540=VERTEX_POINT('',#6633);
#1541=VERTEX_POINT('',#6634);
#1542=VERTEX_POINT('',#6657);
#1543=VERTEX_POINT('',#6659);
#1544=VERTEX_POINT('',#6664);
#1545=VERTEX_POINT('',#6691);
#1546=VERTEX_POINT('',#6692);
#1547=VERTEX_POINT('',#6694);
#1548=VERTEX_POINT('',#6696);
#1549=VERTEX_POINT('',#6698);
#1550=VERTEX_POINT('',#6700);
#1551=VERTEX_POINT('',#6702);
#1552=VERTEX_POINT('',#6705);
#1553=VERTEX_POINT('',#6707);
#1554=VERTEX_POINT('',#6709);
#1555=VERTEX_POINT('',#6757);
#1556=VERTEX_POINT('',#6783);
#1557=VERTEX_POINT('',#6809);
#1558=VERTEX_POINT('',#6811);
#1559=VERTEX_POINT('',#6815);
#1560=VERTEX_POINT('',#6817);
#1561=VERTEX_POINT('',#6821);
#1562=VERTEX_POINT('',#6825);
#1563=VERTEX_POINT('',#6827);
#1564=VERTEX_POINT('',#6831);
#1565=VERTEX_POINT('',#6833);
#1566=VERTEX_POINT('',#6837);
#1567=VERTEX_POINT('',#6839);
#1878=EDGE_CURVE('',#1535,#1536,#138,.T.);
#1879=EDGE_CURVE('',#1535,#1537,#890,.T.);
#1880=EDGE_CURVE('',#1538,#1537,#139,.F.);
#1881=EDGE_CURVE('',#1539,#1538,#140,.F.);
#1882=EDGE_CURVE('',#1536,#1539,#891,.T.);
#1883=EDGE_CURVE('',#1540,#1541,#141,.T.);
#1884=EDGE_CURVE('',#1540,#1542,#892,.T.);
#1885=EDGE_CURVE('',#1543,#1542,#142,.F.);
#1886=EDGE_CURVE('',#1544,#1543,#143,.F.);
#1887=EDGE_CURVE('',#1541,#1544,#893,.T.);
#1888=EDGE_CURVE('',#1545,#1546,#1197,.T.);
#1889=EDGE_CURVE('',#1546,#1547,#894,.T.);
#1890=EDGE_CURVE('',#1548,#1547,#1198,.T.);
#1891=EDGE_CURVE('',#1548,#1549,#895,.T.);
#1892=EDGE_CURVE('',#1549,#1550,#1199,.T.);
#1893=EDGE_CURVE('',#1550,#1551,#896,.T.);
#1894=EDGE_CURVE('',#1551,#1551,#1200,.T.);
#1895=EDGE_CURVE('',#1550,#1552,#1201,.T.);
#1896=EDGE_CURVE('',#1552,#1553,#897,.T.);
#1897=EDGE_CURVE('',#1554,#1553,#1202,.T.);
#1898=EDGE_CURVE('',#1554,#1545,#898,.T.);
#1899=EDGE_CURVE('',#1536,#1535,#144,.T.);
#1900=EDGE_CURVE('',#1541,#1540,#145,.T.);
#1901=EDGE_CURVE('',#1538,#1555,#899,.T.);
#1902=EDGE_CURVE('',#1555,#1555,#1203,.T.);
#1903=EDGE_CURVE('',#1537,#1539,#146,.T.);
#1904=EDGE_CURVE('',#1556,#1556,#1204,.T.);
#1905=EDGE_CURVE('',#1556,#1543,#900,.T.);
#1906=EDGE_CURVE('',#1542,#1544,#147,.T.);
#1907=EDGE_CURVE('',#1557,#1557,#1205,.T.);
#1908=EDGE_CURVE('',#1557,#1558,#901,.T.);
#1909=EDGE_CURVE('',#1558,#1558,#1206,.T.);
#1910=EDGE_CURVE('',#1559,#1559,#1207,.T.);
#1911=EDGE_CURVE('',#1559,#1560,#902,.T.);
#1912=EDGE_CURVE('',#1560,#1560,#1208,.T.);
#1913=EDGE_CURVE('',#1561,#1561,#1209,.T.);
#1914=EDGE_CURVE('',#1561,#1559,#903,.T.);
#1915=EDGE_CURVE('',#1562,#1562,#1210,.T.);
#1916=EDGE_CURVE('',#1562,#1563,#904,.T.);
#1917=EDGE_CURVE('',#1563,#1563,#1211,.T.);
#1918=EDGE_CURVE('',#1564,#1564,#1212,.T.);
#1919=EDGE_CURVE('',#1564,#1565,#905,.T.);
#1920=EDGE_CURVE('',#1565,#1565,#1213,.T.);
#1921=EDGE_CURVE('',#1566,#1566,#1214,.T.);
#1922=EDGE_CURVE('',#1566,#1567,#906,.T.);
#1923=EDGE_CURVE('',#1567,#1567,#1215,.T.);
#1924=EDGE_CURVE('',#1554,#1553,#907,.T.);
#1925=EDGE_CURVE('',#1545,#1552,#908,.T.);
#1926=EDGE_CURVE('',#1546,#1549,#909,.T.);
#1927=EDGE_CURVE('',#1547,#1548,#910,.T.);
#2530=ORIENTED_EDGE('',*,*,#1878,.F.);
#2531=ORIENTED_EDGE('',*,*,#1879,.T.);
#2532=ORIENTED_EDGE('',*,*,#1880,.F.);
#2533=ORIENTED_EDGE('',*,*,#1881,.F.);
#2534=ORIENTED_EDGE('',*,*,#1882,.F.);
#2535=ORIENTED_EDGE('',*,*,#1883,.F.);
#2536=ORIENTED_EDGE('',*,*,#1884,.T.);
#2537=ORIENTED_EDGE('',*,*,#1885,.F.);
#2538=ORIENTED_EDGE('',*,*,#1886,.F.);
#2539=ORIENTED_EDGE('',*,*,#1887,.F.);
#2540=ORIENTED_EDGE('',*,*,#1888,.T.);
#2541=ORIENTED_EDGE('',*,*,#1889,.T.);
#2542=ORIENTED_EDGE('',*,*,#1890,.F.);
#2543=ORIENTED_EDGE('',*,*,#1891,.T.);
#2544=ORIENTED_EDGE('',*,*,#1892,.T.);
#2545=ORIENTED_EDGE('',*,*,#1893,.T.);
#2546=ORIENTED_EDGE('',*,*,#1894,.F.);
#2547=ORIENTED_EDGE('',*,*,#1893,.F.);
#2548=ORIENTED_EDGE('',*,*,#1895,.T.);
#2549=ORIENTED_EDGE('',*,*,#1896,.T.);
#2550=ORIENTED_EDGE('',*,*,#1897,.F.);
#2551=ORIENTED_EDGE('',*,*,#1898,.T.);
#2552=ORIENTED_EDGE('',*,*,#1899,.T.);
#2553=ORIENTED_EDGE('',*,*,#1878,.T.);
#2554=ORIENTED_EDGE('',*,*,#1900,.T.);
#2555=ORIENTED_EDGE('',*,*,#1883,.T.);
#2556=ORIENTED_EDGE('',*,*,#1881,.T.);
#2557=ORIENTED_EDGE('',*,*,#1901,.T.);
#2558=ORIENTED_EDGE('',*,*,#1902,.F.);
#2559=ORIENTED_EDGE('',*,*,#1901,.F.);
#2560=ORIENTED_EDGE('',*,*,#1880,.T.);
#2561=ORIENTED_EDGE('',*,*,#1903,.T.);
#2562=ORIENTED_EDGE('',*,*,#1904,.F.);
#2563=ORIENTED_EDGE('',*,*,#1905,.T.);
#2564=ORIENTED_EDGE('',*,*,#1885,.T.);
#2565=ORIENTED_EDGE('',*,*,#1906,.T.);
#2566=ORIENTED_EDGE('',*,*,#1886,.T.);
#2567=ORIENTED_EDGE('',*,*,#1905,.F.);
#2568=ORIENTED_EDGE('',*,*,#1907,.F.);
#2569=ORIENTED_EDGE('',*,*,#1908,.T.);
#2570=ORIENTED_EDGE('',*,*,#1909,.T.);
#2571=ORIENTED_EDGE('',*,*,#1908,.F.);
#2572=ORIENTED_EDGE('',*,*,#1910,.F.);
#2573=ORIENTED_EDGE('',*,*,#1911,.T.);
#2574=ORIENTED_EDGE('',*,*,#1912,.F.);
#2575=ORIENTED_EDGE('',*,*,#1911,.F.);
#2576=ORIENTED_EDGE('',*,*,#1913,.F.);
#2577=ORIENTED_EDGE('',*,*,#1914,.T.);
#2578=ORIENTED_EDGE('',*,*,#1910,.T.);
#2579=ORIENTED_EDGE('',*,*,#1914,.F.);
#2580=ORIENTED_EDGE('',*,*,#1915,.F.);
#2581=ORIENTED_EDGE('',*,*,#1916,.T.);
#2582=ORIENTED_EDGE('',*,*,#1917,.T.);
#2583=ORIENTED_EDGE('',*,*,#1916,.F.);
#2584=ORIENTED_EDGE('',*,*,#1918,.F.);
#2585=ORIENTED_EDGE('',*,*,#1919,.T.);
#2586=ORIENTED_EDGE('',*,*,#1920,.T.);
#2587=ORIENTED_EDGE('',*,*,#1919,.F.);
#2588=ORIENTED_EDGE('',*,*,#1921,.T.);
#2589=ORIENTED_EDGE('',*,*,#1922,.T.);
#2590=ORIENTED_EDGE('',*,*,#1923,.T.);
#2591=ORIENTED_EDGE('',*,*,#1922,.F.);
#2592=ORIENTED_EDGE('',*,*,#1923,.F.);
#2593=ORIENTED_EDGE('',*,*,#1918,.T.);
#2594=ORIENTED_EDGE('',*,*,#1920,.F.);
#2595=ORIENTED_EDGE('',*,*,#1915,.T.);
#2596=ORIENTED_EDGE('',*,*,#1917,.F.);
#2597=ORIENTED_EDGE('',*,*,#1913,.T.);
#2598=ORIENTED_EDGE('',*,*,#1912,.T.);
#2599=ORIENTED_EDGE('',*,*,#1894,.T.);
#2600=ORIENTED_EDGE('',*,*,#1909,.F.);
#2601=ORIENTED_EDGE('',*,*,#1921,.F.);
#2602=ORIENTED_EDGE('',*,*,#1907,.T.);
#2603=ORIENTED_EDGE('',*,*,#1884,.F.);
#2604=ORIENTED_EDGE('',*,*,#1900,.F.);
#2605=ORIENTED_EDGE('',*,*,#1887,.T.);
#2606=ORIENTED_EDGE('',*,*,#1906,.F.);
#2607=ORIENTED_EDGE('',*,*,#1879,.F.);
#2608=ORIENTED_EDGE('',*,*,#1899,.F.);
#2609=ORIENTED_EDGE('',*,*,#1882,.T.);
#2610=ORIENTED_EDGE('',*,*,#1903,.F.);
#2611=ORIENTED_EDGE('',*,*,#1897,.T.);
#2612=ORIENTED_EDGE('',*,*,#1924,.F.);
#2613=ORIENTED_EDGE('',*,*,#1925,.F.);
#2614=ORIENTED_EDGE('',*,*,#1898,.F.);
#2615=ORIENTED_EDGE('',*,*,#1924,.T.);
#2616=ORIENTED_EDGE('',*,*,#1896,.F.);
#2617=ORIENTED_EDGE('',*,*,#1904,.T.);
#2618=ORIENTED_EDGE('',*,*,#1926,.F.);
#2619=ORIENTED_EDGE('',*,*,#1888,.F.);
#2620=ORIENTED_EDGE('',*,*,#1925,.T.);
#2621=ORIENTED_EDGE('',*,*,#1895,.F.);
#2622=ORIENTED_EDGE('',*,*,#1892,.F.);
#2623=ORIENTED_EDGE('',*,*,#1926,.T.);
#2624=ORIENTED_EDGE('',*,*,#1891,.F.);
#2625=ORIENTED_EDGE('',*,*,#1927,.F.);
#2626=ORIENTED_EDGE('',*,*,#1889,.F.);
#2627=ORIENTED_EDGE('',*,*,#1902,.T.);
#2628=ORIENTED_EDGE('',*,*,#1890,.T.);
#2629=ORIENTED_EDGE('',*,*,#1927,.T.);
#3171=CYLINDRICAL_SURFACE('',#3652,3.);
#3172=CYLINDRICAL_SURFACE('',#3659,1.);
#3173=CYLINDRICAL_SURFACE('',#3661,1.);
#3174=CYLINDRICAL_SURFACE('',#3663,2.3);
#3175=CYLINDRICAL_SURFACE('',#3669,1.14999999999999);
#3176=CYLINDRICAL_SURFACE('',#3671,1.49999999999999);
#3177=CYLINDRICAL_SURFACE('',#3677,3.);
#3274=ADVANCED_FACE('',(#362),#155,.T.);
#3275=ADVANCED_FACE('',(#363),#156,.T.);
#3276=ADVANCED_FACE('',(#364,#212,#213),#3171,.T.);
#3277=ADVANCED_FACE('',(#365),#3172,.F.);
#3278=ADVANCED_FACE('',(#366),#3173,.F.);
#3279=ADVANCED_FACE('',(#367),#3174,.T.);
#3280=ADVANCED_FACE('',(#368),#135,.T.);
#3281=ADVANCED_FACE('',(#369),#3175,.T.);
#3282=ADVANCED_FACE('',(#370),#3176,.T.);
#3283=ADVANCED_FACE('',(#371),#136,.T.);
#3284=ADVANCED_FACE('',(#372),#3177,.T.);
#3285=ADVANCED_FACE('',(#373,#214),#271,.F.);
#3286=ADVANCED_FACE('',(#374,#215),#272,.F.);
#3287=ADVANCED_FACE('',(#375,#216),#273,.F.);
#3288=ADVANCED_FACE('',(#376),#274,.F.);
#3289=ADVANCED_FACE('',(#377,#217),#275,.T.);
#3290=ADVANCED_FACE('',(#378,#218),#276,.T.);
#3291=ADVANCED_FACE('',(#379),#157,.T.);
#3292=ADVANCED_FACE('',(#380),#158,.T.);
#3293=ADVANCED_FACE('',(#381),#277,.F.);
#3294=ADVANCED_FACE('',(#382,#219),#278,.F.);
#3295=ADVANCED_FACE('',(#383),#279,.F.);
#3296=ADVANCED_FACE('',(#384,#220),#280,.F.);
#3297=ADVANCED_FACE('',(#385),#281,.F.);
#3430=CLOSED_SHELL('',(#3274,#3275,#3276,#3277,#3278,#3279,#3280,#3281,
#3282,#3283,#3284,#3285,#3286,#3287,#3288,#3289,#3290,#3291,#3292,#3293,
#3294,#3295,#3296,#3297));
#3651=AXIS2_PLACEMENT_3D('',#5591,#4395,#4396);
#3652=AXIS2_PLACEMENT_3D('',#6690,#4401,#4402);
#3653=AXIS2_PLACEMENT_3D('',#6693,#4403,#4404);
#3654=AXIS2_PLACEMENT_3D('',#6697,#4406,#4407);
#3655=AXIS2_PLACEMENT_3D('',#6701,#4409,#4410);
#3656=AXIS2_PLACEMENT_3D('',#6704,#4412,#4413);
#3657=AXIS2_PLACEMENT_3D('',#6706,#4414,#4415);
#3658=AXIS2_PLACEMENT_3D('',#6710,#4417,#4418);
#3659=AXIS2_PLACEMENT_3D('',#6756,#4420,#4421);
#3660=AXIS2_PLACEMENT_3D('',#6759,#4423,#4424);
#3661=AXIS2_PLACEMENT_3D('',#6782,#4425,#4426);
#3662=AXIS2_PLACEMENT_3D('',#6784,#4427,#4428);
#3663=AXIS2_PLACEMENT_3D('',#6808,#4430,#4431);
#3664=AXIS2_PLACEMENT_3D('',#6810,#4432,#4433);
#3665=AXIS2_PLACEMENT_3D('',#6813,#4435,#4436);
#3666=AXIS2_PLACEMENT_3D('',#6814,#4437,#4438);
#3667=AXIS2_PLACEMENT_3D('',#6816,#4439,#4440);
#3668=AXIS2_PLACEMENT_3D('',#6819,#4442,#4443);
#3669=AXIS2_PLACEMENT_3D('',#6820,#4444,#4445);
#3670=AXIS2_PLACEMENT_3D('',#6822,#4446,#4447);
#3671=AXIS2_PLACEMENT_3D('',#6824,#4449,#4450);
#3672=AXIS2_PLACEMENT_3D('',#6826,#4451,#4452);
#3673=AXIS2_PLACEMENT_3D('',#6829,#4454,#4455);
#3674=AXIS2_PLACEMENT_3D('',#6830,#4456,#4457);
#3675=AXIS2_PLACEMENT_3D('',#6832,#4458,#4459);
#3676=AXIS2_PLACEMENT_3D('',#6835,#4461,#4462);
#3677=AXIS2_PLACEMENT_3D('',#6836,#4463,#4464);
#3678=AXIS2_PLACEMENT_3D('',#6838,#4465,#4466);
#3679=AXIS2_PLACEMENT_3D('',#6841,#4468,#4469);
#3680=AXIS2_PLACEMENT_3D('',#6842,#4470,#4471);
#3681=AXIS2_PLACEMENT_3D('',#6843,#4472,#4473);
#3682=AXIS2_PLACEMENT_3D('',#6844,#4474,#4475);
#3683=AXIS2_PLACEMENT_3D('',#6845,#4476,#4477);
#3684=AXIS2_PLACEMENT_3D('',#6846,#4478,#4479);
#3685=AXIS2_PLACEMENT_3D('',#6847,#4480,#4481);
#3686=AXIS2_PLACEMENT_3D('',#7832,#4482,#4483);
#3687=AXIS2_PLACEMENT_3D('',#7834,#4485,#4486);
#3688=AXIS2_PLACEMENT_3D('',#7836,#4488,#4489);
#3689=AXIS2_PLACEMENT_3D('',#7838,#4491,#4492);
#3690=AXIS2_PLACEMENT_3D('',#7840,#4494,#4495);
#4395=DIRECTION('axis',(0.,0.,1.));
#4396=DIRECTION('refdir',(1.,0.,0.));
#4397=DIRECTION('',(0.404889385483999,-6.75715337925259E-5,0.914365671357186));
#4398=DIRECTION('',(-0.404889387332683,-2.14111170223934E-15,0.914365673035337));
#4399=DIRECTION('',(0.404889385483998,6.75715337926642E-5,-0.914365671357186));
#4400=DIRECTION('',(-0.404889387332682,4.97544927214364E-16,-0.914365673035337));
#4401=DIRECTION('center_axis',(-1.,-1.83084271870903E-16,0.));
#4402=DIRECTION('ref_axis',(1.83084271870903E-16,-1.,0.));
#4403=DIRECTION('center_axis',(1.,0.,0.));
#4404=DIRECTION('ref_axis',(0.,0.,-1.));
#4405=DIRECTION('',(-1.,-1.83084271870903E-16,0.));
#4406=DIRECTION('center_axis',(-1.,-1.83084271870903E-16,0.));
#4407=DIRECTION('ref_axis',(1.83084271870903E-16,-1.,0.));
#4408=DIRECTION('',(1.,1.83084271870903E-16,0.));
#4409=DIRECTION('center_axis',(1.,0.,0.));
#4410=DIRECTION('ref_axis',(0.,0.,-1.));
#4411=DIRECTION('',(1.,1.83084271870903E-16,0.));
#4412=DIRECTION('center_axis',(1.,-4.57710679677258E-17,0.));
#4413=DIRECTION('ref_axis',(4.57710679677258E-17,1.,0.));
#4414=DIRECTION('center_axis',(1.,0.,0.));
#4415=DIRECTION('ref_axis',(0.,0.,-1.));
#4416=DIRECTION('',(-1.,-1.83084271870903E-16,0.));
#4417=DIRECTION('center_axis',(-1.,-1.83084271870903E-16,0.));
#4418=DIRECTION('ref_axis',(1.83084271870903E-16,-1.,0.));
#4419=DIRECTION('',(1.,1.83084271870903E-16,0.));
#4420=DIRECTION('center_axis',(0.,0.,1.));
#4421=DIRECTION('ref_axis',(1.,0.,0.));
#4422=DIRECTION('',(0.,0.,1.));
#4423=DIRECTION('center_axis',(0.,0.,-1.));
#4424=DIRECTION('ref_axis',(-1.,0.,0.));
#4425=DIRECTION('center_axis',(0.,0.,1.));
#4426=DIRECTION('ref_axis',(1.,0.,0.));
#4427=DIRECTION('center_axis',(1.42580011724121E-15,0.,1.));
#4428=DIRECTION('ref_axis',(1.,0.,-1.42580011724121E-15));
#4429=DIRECTION('',(0.,0.,1.));
#4430=DIRECTION('center_axis',(1.,-4.57710679677258E-17,0.));
#4431=DIRECTION('ref_axis',(4.57710679677258E-17,1.,0.));
#4432=DIRECTION('center_axis',(1.,-4.57710679677258E-17,0.));
#4433=DIRECTION('ref_axis',(4.57710679677258E-17,1.,0.));
#4434=DIRECTION('',(-1.,4.57710679677258E-17,0.));
#4435=DIRECTION('center_axis',(1.,-4.57710679677258E-17,0.));
#4436=DIRECTION('ref_axis',(4.57710679677258E-17,1.,0.));
#4437=DIRECTION('center_axis',(-1.,-1.83084271870902E-16,0.));
#4438=DIRECTION('ref_axis',(1.83084271870902E-16,-1.,0.));
#4439=DIRECTION('center_axis',(-1.,-1.83084271870902E-16,0.));
#4440=DIRECTION('ref_axis',(1.83084271870902E-16,-1.,0.));
#4441=DIRECTION('',(0.707106781186537,-0.707106781186558,8.65956056235506E-17));
#4442=DIRECTION('center_axis',(1.,1.83084271870903E-16,0.));
#4443=DIRECTION('ref_axis',(1.83084271870903E-16,-1.,0.));
#4444=DIRECTION('center_axis',(-1.,-1.83084271870903E-16,0.));
#4445=DIRECTION('ref_axis',(1.83084271870903E-16,-1.,0.));
#4446=DIRECTION('center_axis',(-1.,-1.83084271870903E-16,0.));
#4447=DIRECTION('ref_axis',(1.83084271870903E-16,-1.,0.));
#4448=DIRECTION('',(1.,1.83084271870903E-16,0.));
#4449=DIRECTION('center_axis',(-1.,-1.83084271870903E-16,0.));
#4450=DIRECTION('ref_axis',(1.83084271870903E-16,-1.,0.));
#4451=DIRECTION('center_axis',(-1.,-1.83084271870903E-16,0.));
#4452=DIRECTION('ref_axis',(1.83084271870903E-16,-1.,0.));
#4453=DIRECTION('',(1.,1.83084271870903E-16,0.));
#4454=DIRECTION('center_axis',(-1.,-1.83084271870903E-16,0.));
#4455=DIRECTION('ref_axis',(1.83084271870903E-16,-1.,0.));
#4456=DIRECTION('center_axis',(-1.,-1.83084271870903E-16,0.));
#4457=DIRECTION('ref_axis',(1.83084271870903E-16,-1.,0.));
#4458=DIRECTION('center_axis',(-1.,-1.83084271870903E-16,0.));
#4459=DIRECTION('ref_axis',(1.83084271870903E-16,-1.,0.));
#4460=DIRECTION('',(0.99522852511998,-0.0975714240313706,1.19490532128267E-17));
#4461=DIRECTION('center_axis',(-1.,-1.83084271870903E-16,0.));
#4462=DIRECTION('ref_axis',(1.83084271870903E-16,-1.,0.));
#4463=DIRECTION('center_axis',(-1.,-1.83084271870903E-16,0.));
#4464=DIRECTION('ref_axis',(1.83084271870903E-16,-1.,0.));
#4465=DIRECTION('center_axis',(1.,-4.57710679677258E-17,0.));
#4466=DIRECTION('ref_axis',(4.57710679677258E-17,1.,0.));
#4467=DIRECTION('',(1.,1.83084271870903E-16,0.));
#4468=DIRECTION('center_axis',(-1.,-1.83084271870903E-16,0.));
#4469=DIRECTION('ref_axis',(1.83084271870903E-16,-1.,0.));
#4470=DIRECTION('center_axis',(-1.,-1.83084271870903E-16,0.));
#4471=DIRECTION('ref_axis',(1.83084271870903E-16,-1.,0.));
#4472=DIRECTION('center_axis',(-1.,-1.83084271870903E-16,0.));
#4473=DIRECTION('ref_axis',(1.83084271870903E-16,-1.,0.));
#4474=DIRECTION('center_axis',(-1.,-1.83084271870903E-16,0.));
#4475=DIRECTION('ref_axis',(1.83084271870903E-16,-1.,0.));
#4476=DIRECTION('center_axis',(-1.,-1.83084271870903E-16,0.));
#4477=DIRECTION('ref_axis',(1.83084271870903E-16,-1.,0.));
#4478=DIRECTION('center_axis',(1.,-4.57710679677258E-17,0.));
#4479=DIRECTION('ref_axis',(4.57710679677258E-17,1.,0.));
#4480=DIRECTION('center_axis',(-1.,4.57710679677258E-17,0.));
#4481=DIRECTION('ref_axis',(-4.57710679677258E-17,-1.,0.));
#4482=DIRECTION('center_axis',(1.,1.83084271870903E-16,0.));
#4483=DIRECTION('ref_axis',(-1.83084271870903E-16,1.,0.));
#4484=DIRECTION('',(0.,1.,0.));
#4485=DIRECTION('center_axis',(1.42580011724121E-15,0.,1.));
#4486=DIRECTION('ref_axis',(1.,0.,-1.42580011724121E-15));
#4487=DIRECTION('',(0.,1.,0.));
#4488=DIRECTION('center_axis',(1.,0.,0.));
#4489=DIRECTION('ref_axis',(0.,0.,-1.));
#4490=DIRECTION('',(0.,1.,0.));
#4491=DIRECTION('center_axis',(0.,0.,-1.));
#4492=DIRECTION('ref_axis',(-1.,0.,0.));
#4493=DIRECTION('',(0.,1.,0.));
#4494=DIRECTION('center_axis',(1.,1.83084271870903E-16,0.));
#4495=DIRECTION('ref_axis',(-1.83084271870903E-16,1.,0.));
#5591=CARTESIAN_POINT('',(0.,0.,0.));
#5592=CARTESIAN_POINT('Ctrl Pts',(-24.7512205732181,1.27647900817359E-15,
-3.00000039251396));
#5593=CARTESIAN_POINT('Ctrl Pts',(-24.7512209918384,0.0224904489448925,
-3.0000001742556));
#5594=CARTESIAN_POINT('Ctrl Pts',(-24.7517089574441,0.0449130845232472,
-2.99974733834206));
#5595=CARTESIAN_POINT('Ctrl Pts',(-24.7536443519837,0.0895752381506401,
-2.99874599882651));
#5596=CARTESIAN_POINT('Ctrl Pts',(-24.7550914179306,0.111823200513364,-2.9979976955573));
#5597=CARTESIAN_POINT('Ctrl Pts',(-24.7608544959128,0.178320919528196,-2.99502476849759));
#5598=CARTESIAN_POINT('Ctrl Pts',(-24.766591932863,0.222335186723984,-2.99207096785045));
#5599=CARTESIAN_POINT('Ctrl Pts',(-24.7780291872986,0.28783719851668,-2.98624078109656));
#5600=CARTESIAN_POINT('Ctrl Pts',(-24.7823200974485,0.309606387247319,-2.98406110217343));
#5601=CARTESIAN_POINT('Ctrl Pts',(-24.789468342319,0.342109605994458,-2.98045008409494));
#5602=CARTESIAN_POINT('Ctrl Pts',(-24.7919728029526,0.352929856681449,-2.97918798270958));
#5603=CARTESIAN_POINT('Ctrl Pts',(-24.7972217651647,0.374523130101453,-2.97655057002885));
#5604=CARTESIAN_POINT('Ctrl Pts',(-24.7999685317995,0.3853026801014,-2.97517414639763));
#5605=CARTESIAN_POINT('Ctrl Pts',(-24.8085250872429,0.417396090242857,-2.97090016875934));
#5606=CARTESIAN_POINT('Ctrl Pts',(-24.81466151752,0.438519418189055,-2.96785256118554));
#5607=CARTESIAN_POINT('Ctrl Pts',(-24.8277811472732,0.480245335622271,-2.96138693176614));
#5608=CARTESIAN_POINT('Ctrl Pts',(-24.8347637590013,0.500846703560909,-2.95796918269451));
#5609=CARTESIAN_POINT('Ctrl Pts',(-24.8569589172265,0.561884990270977,-2.94720128262928));
#5610=CARTESIAN_POINT('Ctrl Pts',(-24.8734161226417,0.601558077547724,-2.93933624108072));
#5611=CARTESIAN_POINT('Ctrl Pts',(-24.9005702937365,0.659577575494014,-2.92666224804854));
#5612=CARTESIAN_POINT('Ctrl Pts',(-24.9100346262345,0.678669948505798,-2.92229102401349));
#5613=CARTESIAN_POINT('Ctrl Pts',(-24.9297928233973,0.716355649282148,-2.91328208432799));
#5614=CARTESIAN_POINT('Ctrl Pts',(-24.9400945131254,0.734962441112191,-2.90864084409791));
#5615=CARTESIAN_POINT('Ctrl Pts',(-24.961514660095,0.771629674000388,-2.89912896911718));
#5616=CARTESIAN_POINT('Ctrl Pts',(-24.9725545674253,0.789557946478682,-2.89429319601545));
#5617=CARTESIAN_POINT('Ctrl Pts',(-24.9953084665056,0.824674949037349,-2.88448368582705));
#5618=CARTESIAN_POINT('Ctrl Pts',(-25.0070179507415,0.84185585681256,-2.87951192539658));
#5619=CARTESIAN_POINT('Ctrl Pts',(-25.043133571216,0.892292847196555,-2.86444548622589));
#5620=CARTESIAN_POINT('Ctrl Pts',(-25.0685243392037,0.924445728200641,-2.85419906644615));
#5621=CARTESIAN_POINT('Ctrl Pts',(-25.1085920152708,0.970518787083059,-2.83872479371572));
#5622=CARTESIAN_POINT('Ctrl Pts',(-25.1222787941031,0.985516398208715,-2.83354919922537));
#5623=CARTESIAN_POINT('Ctrl Pts',(-25.1503247573348,1.0147909893251,-2.82319728666854));
#5624=CARTESIAN_POINT('Ctrl Pts',(-25.164690788982,1.02907375849125,-2.81801865872126));
#5625=CARTESIAN_POINT('Ctrl Pts',(-25.1940841805899,1.05688925756545,-2.80770519124119));
#5626=CARTESIAN_POINT('Ctrl Pts',(-25.2091790647757,1.07047808243068,-2.80254833483865));
#5627=CARTESIAN_POINT('Ctrl Pts',(-25.2397860183817,1.09666813400314,-2.79240366726727));
#5628=CARTESIAN_POINT('Ctrl Pts',(-25.2553204379955,1.10929595959291,-2.78740689519964));
#5629=CARTESIAN_POINT('Ctrl Pts',(-25.2868471218303,1.13362876731756,-2.77759978805859));
#5630=CARTESIAN_POINT('Ctrl Pts',(-25.3028398226619,1.14533472511361,-2.77278915814534));
#5631=CARTESIAN_POINT('Ctrl Pts',(-25.3352862383422,1.16783527307202,-2.76338780408879));
#5632=CARTESIAN_POINT('Ctrl Pts',(-25.351739959153,1.17862983581217,-2.75879704618161));
#5633=CARTESIAN_POINT('Ctrl Pts',(-25.4018015943325,1.20964925021434,-2.74540688876098));
#5634=CARTESIAN_POINT('Ctrl Pts',(-25.4361159534219,1.22851653432306,-2.73698721829837));
#5635=CARTESIAN_POINT('Ctrl Pts',(-25.4890321005069,1.25402677583021,-2.72534532216722));
#5636=CARTESIAN_POINT('Ctrl Pts',(-25.5069295704027,1.26207047477093,-2.72162643380116));
#5637=CARTESIAN_POINT('Ctrl Pts',(-25.5341342320122,1.27341408145951,-2.71632781873948));
#5638=CARTESIAN_POINT('Ctrl Pts',(-25.5432728261675,1.27707857798257,-2.71460649012167));
#5639=CARTESIAN_POINT('Ctrl Pts',(-25.5616697300355,1.28416247287641,-2.71126260047886));
#5640=CARTESIAN_POINT('Ctrl Pts',(-25.5709428123064,1.28758661927442,-2.70963775628573));
#5641=CARTESIAN_POINT('Ctrl Pts',(-25.5987921995341,1.29743171221407,-2.70494481626589));
#5642=CARTESIAN_POINT('Ctrl Pts',(-25.6174339809943,1.30344290404711,-2.70205039524381));
#5643=CARTESIAN_POINT('Ctrl Pts',(-25.6548880488268,1.31438298806205,-2.69674565415259));
#5644=CARTESIAN_POINT('Ctrl Pts',(-25.6736969296858,1.31931098956043,-2.69433575157957));
#5645=CARTESIAN_POINT('Ctrl Pts',(-25.7303690862317,1.33248199267998,-2.68785983771893));
#5646=CARTESIAN_POINT('Ctrl Pts',(-25.7684774334826,1.33911568210638,-2.68454786410377));
#5647=CARTESIAN_POINT('Ctrl Pts',(-25.8261391530629,1.34582335222857,-2.6811878846237));
#5648=CARTESIAN_POINT('Ctrl Pts',(-25.8454430323917,1.34751786899547,-2.68033581181979));
#5649=CARTESIAN_POINT('Ctrl Pts',(-25.8842203925786,1.34980777647362,-2.67918335088873));
#5650=CARTESIAN_POINT('Ctrl Pts',(-25.903705143976,1.35040245497256,-2.67888335709824));
#5651=CARTESIAN_POINT('Ctrl Pts',(-25.9428031383705,1.3504709734195,-2.67884881443484));
#5652=CARTESIAN_POINT('Ctrl Pts',(-25.9625262668505,1.34993687451434,-2.67911827983487));
#5653=CARTESIAN_POINT('Ctrl Pts',(-26.0016751544635,1.34774181046255,-2.68022319148998));
#5654=CARTESIAN_POINT('Ctrl Pts',(-26.0211401155725,1.34608678179489,-2.68105562372842));
#5655=CARTESIAN_POINT('Ctrl Pts',(-26.059852112923,1.3416829898099,-2.68326212736971));
#5656=CARTESIAN_POINT('Ctrl Pts',(-26.0790998997345,1.33893483082381,-2.68463587910205));
#5657=CARTESIAN_POINT('Ctrl Pts',(-26.1173832113779,1.33236210276061,-2.6879039252919));
#5658=CARTESIAN_POINT('Ctrl Pts',(-26.1364187282489,1.32853748653122,-2.6897982252467));
#5659=CARTESIAN_POINT('Ctrl Pts',(-26.1932111473027,1.31546058553579,-2.69623084419525));
#5660=CARTESIAN_POINT('Ctrl Pts',(-26.2306587701737,1.30460495425469,-2.70152087608486));
#5661=CARTESIAN_POINT('Ctrl Pts',(-26.2769393229609,1.2883550701772,-2.70927245589677));
#5662=CARTESIAN_POINT('Ctrl Pts',(-26.2861735714613,1.28496732277494,-2.7108812019877));
#5663=CARTESIAN_POINT('Ctrl Pts',(-26.3045800008344,1.27792560939945,-2.71420782302654));
#5664=CARTESIAN_POINT('Ctrl Pts',(-26.3137695365298,1.27426364167248,-2.71592937831152));
#5665=CARTESIAN_POINT('Ctrl Pts',(-26.3411342135086,1.26291934373526,-2.72123265364053));
#5666=CARTESIAN_POINT('Ctrl Pts',(-26.359108489593,1.25488165967843,-2.72495179584751));
#5667=CARTESIAN_POINT('Ctrl Pts',(-26.3945729485002,1.23786371810423,-2.73272458713573));
#5668=CARTESIAN_POINT('Ctrl Pts',(-26.4120572689161,1.2288861049134,-2.73677701321045));
#5669=CARTESIAN_POINT('Ctrl Pts',(-26.4465442238038,1.21000802381103,-2.74517577574545));
#5670=CARTESIAN_POINT('Ctrl Pts',(-26.4635468416443,1.20010753017732,-2.74952213668882));
#5671=CARTESIAN_POINT('Ctrl Pts',(-26.4970804298005,1.17938992628659,-2.75847230162352));
#5672=CARTESIAN_POINT('Ctrl Pts',(-26.5136113919084,1.16857280798543,-2.76307612855274));
#5673=CARTESIAN_POINT('Ctrl Pts',(-26.5462078840406,1.14602038731631,-2.77250596727388));
#5674=CARTESIAN_POINT('Ctrl Pts',(-26.562273493867,1.1342850254395,-2.77733202823839));
#5675=CARTESIAN_POINT('Ctrl Pts',(-26.5939414283119,1.10988700911992,-2.78717177677759));
#5676=CARTESIAN_POINT('Ctrl Pts',(-26.6095473445415,1.09722131473956,-2.79218666030943));
#5677=CARTESIAN_POINT('Ctrl Pts',(-26.6402811143626,1.0709566148845,-2.8023656091679));
#5678=CARTESIAN_POINT('Ctrl Pts',(-26.6552948463125,1.05745575069761,-2.80749156457345));
#5679=CARTESIAN_POINT('Ctrl Pts',(-26.6846546110444,1.02971343125002,-2.817784903976));
#5680=CARTESIAN_POINT('Ctrl Pts',(-26.6989977054847,1.0154744409772,-2.82295134426973));
#5681=CARTESIAN_POINT('Ctrl Pts',(-26.7270250638549,0.986265666309434,-2.83328830718171));
#5682=CARTESIAN_POINT('Ctrl Pts',(-26.7407092830319,0.971295850373597,-2.83845888576662));
#5683=CARTESIAN_POINT('Ctrl Pts',(-26.7807869864753,0.925288343298038,-2.85392552592912));
#5684=CARTESIAN_POINT('Ctrl Pts',(-26.8062104528913,0.893151438987838,-2.86417785822885));
#5685=CARTESIAN_POINT('Ctrl Pts',(-26.8423944800688,0.842704105273585,-2.87926390500452));
#5686=CARTESIAN_POINT('Ctrl Pts',(-26.854135591242,0.825504489114966,-2.88424645343755));
#5687=CARTESIAN_POINT('Ctrl Pts',(-26.8712462612575,0.799138658144538,-2.89161951102431));
#5688=CARTESIAN_POINT('Ctrl Pts',(-26.876870779104,0.790247883055742,-2.89406240563576));
#5689=CARTESIAN_POINT('Ctrl Pts',(-26.8879469072247,0.772281655830631,-2.89890846334945));
#5690=CARTESIAN_POINT('Ctrl Pts',(-26.893409269784,0.763187520111317,-2.90131641792487));
#5691=CARTESIAN_POINT('Ctrl Pts',(-26.9094749238114,0.735724555729973,-2.90844791977076));
#5692=CARTESIAN_POINT('Ctrl Pts',(-26.9197549867311,0.717184843056236,-2.91307769758814));
#5693=CARTESIAN_POINT('Ctrl Pts',(-26.9394913365264,0.679605859000127,-2.92207317082987));
#5694=CARTESIAN_POINT('Ctrl Pts',(-26.9489438557812,0.66057330364731,-2.92643722327291));
#5695=CARTESIAN_POINT('Ctrl Pts',(-26.9760661551845,0.602745633656238,-2.93909124911831));
#5696=CARTESIAN_POINT('Ctrl Pts',(-26.9925036507446,0.563222175536771,-2.94694362837257));
#5697=CARTESIAN_POINT('Ctrl Pts',(-27.0220715762404,0.482184664459273,-2.96128235245645));
#5698=CARTESIAN_POINT('Ctrl Pts',(-27.0352035249924,0.440658030285019,-2.96777002657));
#5699=CARTESIAN_POINT('Ctrl Pts',(-27.0523216883035,0.376833839229868,-2.97631699067074));
#5700=CARTESIAN_POINT('Ctrl Pts',(-27.0576005303158,0.355274412887374,-2.97897027612798));
#5701=CARTESIAN_POINT('Ctrl Pts',(-27.0672600591522,0.311662753136127,-2.98384821443584));
#5702=CARTESIAN_POINT('Ctrl Pts',(-27.0716114828177,0.289741794867057,-2.9860580250039));
#5703=CARTESIAN_POINT('Ctrl Pts',(-27.0793660357628,0.245626078050727,-2.99001014183973));
#5704=CARTESIAN_POINT('Ctrl Pts',(-27.0827661298392,0.223449095191074,-2.99175090619715));
#5705=CARTESIAN_POINT('Ctrl Pts',(-27.088612570746,0.178789136156299,-2.99475173451271));
#5706=CARTESIAN_POINT('Ctrl Pts',(-27.0910448696872,0.156404671590301,-2.99600458388059));
#5707=CARTESIAN_POINT('Ctrl Pts',(-27.096853679446,0.0893800225646476,-2.9990010619891));
#5708=CARTESIAN_POINT('Ctrl Pts',(-27.098776248484,0.0447217666279721,-2.99999873125252));
#5709=CARTESIAN_POINT('Ctrl Pts',(-27.0987810099015,-0.0221932423036774,
-3.00000122002206));
#5710=CARTESIAN_POINT('Ctrl Pts',(-27.0983026039981,-0.0444881794306497,
-2.99975332625577));
#5711=CARTESIAN_POINT('Ctrl Pts',(-27.0963847740834,-0.0890579105479476,
-2.99876106205554));
#5712=CARTESIAN_POINT('Ctrl Pts',(-27.0949453773136,-0.111332705013248,
-2.99801669216856));
#5713=CARTESIAN_POINT('Ctrl Pts',(-27.0910975380372,-0.155862012281646,
-2.99603172453301));
#5714=CARTESIAN_POINT('Ctrl Pts',(-27.0886879051299,-0.178121225730192,
-2.99479051237394));
#5715=CARTESIAN_POINT('Ctrl Pts',(-27.0828889596371,-0.222600296296536,
-2.99181384430895));
#5716=CARTESIAN_POINT('Ctrl Pts',(-27.0794840506901,-0.24488839674227,-2.99007048023225));
#5717=CARTESIAN_POINT('Ctrl Pts',(-27.071775952777,-0.288869899263924,-2.98614166251469));
#5718=CARTESIAN_POINT('Ctrl Pts',(-27.0674608269688,-0.310670331278561,
-2.98395006519913));
#5719=CARTESIAN_POINT('Ctrl Pts',(-27.0579363802439,-0.353839366034688,
-2.9791394357373));
#5720=CARTESIAN_POINT('Ctrl Pts',(-27.0527258255725,-0.375218389994937,
-2.97651976178012));
#5721=CARTESIAN_POINT('Ctrl Pts',(-27.0357695640527,-0.438751704381787,
-2.96805078583667));
#5722=CARTESIAN_POINT('Ctrl Pts',(-27.0226990393997,-0.480310373169669,
-2.96158999423888));
#5723=CARTESIAN_POINT('Ctrl Pts',(-27.0004754778274,-0.541446390227559,
-2.95080792183841));
#5724=CARTESIAN_POINT('Ctrl Pts',(-26.9926233391618,-0.561639756422953,
-2.94702858491464));
#5725=CARTESIAN_POINT('Ctrl Pts',(-26.9801906409175,-0.591614002592807,
-2.94110512698185));
#5726=CARTESIAN_POINT('Ctrl Pts',(-26.9759329233523,-0.601561926835125,
-2.9390861971729));
#5727=CARTESIAN_POINT('Ctrl Pts',(-26.9671986892834,-0.621350277064196,
-2.93496653895837));
#5728=CARTESIAN_POINT('Ctrl Pts',(-26.9627160190822,-0.63120305480576,-2.932862972483));
#5729=CARTESIAN_POINT('Ctrl Pts',(-26.949000010224,-0.660466243653679,-2.92646286445819));
#5730=CARTESIAN_POINT('Ctrl Pts',(-26.9394863006083,-0.679616625492289,
-2.92207081256717));
#5731=CARTESIAN_POINT('Ctrl Pts',(-26.9197260539462,-0.717238752620477,
-2.91306457362862));
#5732=CARTESIAN_POINT('Ctrl Pts',(-26.9094809907086,-0.735707812001506,
-2.90845102679016));
#5733=CARTESIAN_POINT('Ctrl Pts',(-26.8776648850953,-0.790113953263625,
-2.8943267049494));
#5734=CARTESIAN_POINT('Ctrl Pts',(-26.8550156533739,-0.825052204529002,
-2.88453180649776));
#5735=CARTESIAN_POINT('Ctrl Pts',(-26.8188825262082,-0.875510966128818,
-2.86945837323707));
#5736=CARTESIAN_POINT('Ctrl Pts',(-26.8064775830923,-0.892005171014228,
-2.86437028648305));
#5737=CARTESIAN_POINT('Ctrl Pts',(-26.7809368156929,-0.924343274785419,
-2.85409879125165));
#5738=CARTESIAN_POINT('Ctrl Pts',(-26.767806005017,-0.940181255880803,-2.84891729113089));
#5739=CARTESIAN_POINT('Ctrl Pts',(-26.7475346890206,-0.963464821076124,
-2.84109226874023));
#5740=CARTESIAN_POINT('Ctrl Pts',(-26.7406844898386,-0.971142790692552,
-2.83847640424402));
#5741=CARTESIAN_POINT('Ctrl Pts',(-26.7268665710498,-0.986257223502061,
-2.83326015443131));
#5742=CARTESIAN_POINT('Ctrl Pts',(-26.7198861854429,-0.993708406579362,
-2.83065485672359));
#5743=CARTESIAN_POINT('Ctrl Pts',(-26.6987543184742,-1.01572209996893,-2.82286262012559));
#5744=CARTESIAN_POINT('Ctrl Pts',(-26.6843926989096,-1.02996746343674,-2.81769174714818));
#5745=CARTESIAN_POINT('Ctrl Pts',(-26.6405194665222,-1.07140391340387,-2.80231410558904));
#5746=CARTESIAN_POINT('Ctrl Pts',(-26.6101987968579,-1.09732460419766,-2.79223276559477));
#5747=CARTESIAN_POINT('Ctrl Pts',(-26.5630918828768,-1.13367250400703,-2.77758169296716));
#5748=CARTESIAN_POINT('Ctrl Pts',(-26.5471174957754,-1.14536614557727,-2.77277626806029));
#5749=CARTESIAN_POINT('Ctrl Pts',(-26.514612671107,-1.167903545887,-2.76335903848249));
#5750=CARTESIAN_POINT('Ctrl Pts',(-26.4980822787532,-1.17874735889938,-2.7587471803173));
#5751=CARTESIAN_POINT('Ctrl Pts',(-26.46444880388,-1.19957259205025,-2.74975580028194));
#5752=CARTESIAN_POINT('Ctrl Pts',(-26.4473524929256,-1.20955009125369,-2.74537799392286));
#5753=CARTESIAN_POINT('Ctrl Pts',(-26.4212416835811,-1.22386590602099,-2.73901119026752));
#5754=CARTESIAN_POINT('Ctrl Pts',(-26.4124619953677,-1.22852739949809,-2.73692306012723));
#5755=CARTESIAN_POINT('Ctrl Pts',(-26.3948577516024,-1.23757286419293,-2.73284480288515));
#5756=CARTESIAN_POINT('Ctrl Pts',(-26.3860147393496,-1.24196779569831,-2.73084989444485));
#5757=CARTESIAN_POINT('Ctrl Pts',(-26.3416451282571,-1.26327195668704,-2.72112034953696));
#5758=CARTESIAN_POINT('Ctrl Pts',(-26.3055754632133,-1.27824521948247,-2.71409222828942));
#5759=CARTESIAN_POINT('Ctrl Pts',(-26.2323060083433,-1.30407984829822,-2.70177412725945));
#5760=CARTESIAN_POINT('Ctrl Pts',(-26.1951016228417,-1.31494638090081,-2.69648191406169));
#5761=CARTESIAN_POINT('Ctrl Pts',(-26.1384100565222,-1.32811542764141,-2.69000670173171));
#5762=CARTESIAN_POINT('Ctrl Pts',(-26.1193651709025,-1.33198245867611,-2.68809214937698));
#5763=CARTESIAN_POINT('Ctrl Pts',(-26.0809718351375,-1.33864905018688,-2.68477846139787));
#5764=CARTESIAN_POINT('Ctrl Pts',(-26.0616267046488,-1.34144791557871,-2.68337970984734));
#5765=CARTESIAN_POINT('Ctrl Pts',(-26.0323637266099,-1.34482464575182,-2.68168810040417));
#5766=CARTESIAN_POINT('Ctrl Pts',(-26.0225572452852,-1.34581322849438,-2.68119198692628));
#5767=CARTESIAN_POINT('Ctrl Pts',(-26.0029866629929,-1.34750144912675,-2.68034392500146));
#5768=CARTESIAN_POINT('Ctrl Pts',(-25.993207230682,-1.34820337332278,-2.67999083517031));
#5769=CARTESIAN_POINT('Ctrl Pts',(-25.9639248638171,-1.34988238530038,-2.67914574940456));
#5770=CARTESIAN_POINT('Ctrl Pts',(-25.944430250381,-1.35043878696277,-2.67886501715932));
#5771=CARTESIAN_POINT('Ctrl Pts',(-25.8861245564454,-1.35043705000303,-2.67886596390227));
#5772=CARTESIAN_POINT('Ctrl Pts',(-25.8474104061639,-1.34822092631382,-2.67998650091243));
#5773=CARTESIAN_POINT('Ctrl Pts',(-25.7896109432291,-1.34160967645964,-2.68329876772692));
#5774=CARTESIAN_POINT('Ctrl Pts',(-25.7703875060739,-1.33885738792583,-2.68467452923362));
#5775=CARTESIAN_POINT('Ctrl Pts',(-25.7320267909422,-1.33224993750147,-2.68795954661435));
#5776=CARTESIAN_POINT('Ctrl Pts',(-25.7128830927771,-1.32839290578458,-2.68986973704836));
#5777=CARTESIAN_POINT('Ctrl Pts',(-25.684251825295,-1.32177548884069,-2.69312428914528));
#5778=CARTESIAN_POINT('Ctrl Pts',(-25.6747142093514,-1.31942848978328,-2.69427521202406));
#5779=CARTESIAN_POINT('Ctrl Pts',(-25.6556603366635,-1.31445289803523,-2.69670614956339));
#5780=CARTESIAN_POINT('Ctrl Pts',(-25.6461500334678,-1.31182518416257,-2.69798570492286));
#5781=CARTESIAN_POINT('Ctrl Pts',(-25.6178200674555,-1.30356617188209,-2.70199101363684));
#5782=CARTESIAN_POINT('Ctrl Pts',(-25.5991463885073,-1.29754777172781,-2.70488904077813));
#5783=CARTESIAN_POINT('Ctrl Pts',(-25.5622143033361,-1.28450992377735,-2.711104791713));
#5784=CARTESIAN_POINT('Ctrl Pts',(-25.5439552645306,-1.27749068571576,-2.71442241845669));
#5785=CARTESIAN_POINT('Ctrl Pts',(-25.5078400226815,-1.26246775944475,-2.72144201858098));
#5786=CARTESIAN_POINT('Ctrl Pts',(-25.4899838433394,-1.25446401700334,-2.72514402265192));
#5787=CARTESIAN_POINT('Ctrl Pts',(-25.4370074508209,-1.22898778436132,-2.736775538613));
#5788=CARTESIAN_POINT('Ctrl Pts',(-25.402476169391,-1.21005033530757,-2.74523167785092));
#5789=CARTESIAN_POINT('Ctrl Pts',(-25.3602840547609,-1.18392811236617,-2.7565104471187));
#5790=CARTESIAN_POINT('Ctrl Pts',(-25.3518921545878,-1.17857779567388,-2.75880270804698));
#5791=CARTESIAN_POINT('Ctrl Pts',(-25.33521027166,-1.16763346103173,-2.76345258994632));
#5792=CARTESIAN_POINT('Ctrl Pts',(-25.3269101970962,-1.16203150593469,-2.76581339519711));
#5793=CARTESIAN_POINT('Ctrl Pts',(-25.3022697723606,-1.14492960216067,-2.77295715687364));
#5794=CARTESIAN_POINT('Ctrl Pts',(-25.2861659342133,-1.13312196993095,-2.77780680847141));
#5795=CARTESIAN_POINT('Ctrl Pts',(-25.2545677370148,-1.10869517847092,-2.78764614588441));
#5796=CARTESIAN_POINT('Ctrl Pts',(-25.2390760976615,-1.09607817216592,-2.79263498420857));
#5797=CARTESIAN_POINT('Ctrl Pts',(-25.2086929585038,-1.0700438882078,-2.80271360615569));
#5798=CARTESIAN_POINT('Ctrl Pts',(-25.1938014786094,-1.05662659440153,-2.80780342156984));
#5799=CARTESIAN_POINT('Ctrl Pts',(-25.1646092945331,-1.02899172455792,-2.81804822663801));
#5800=CARTESIAN_POINT('Ctrl Pts',(-25.1503085987059,-1.01477414783797,-2.82320324630944));
#5801=CARTESIAN_POINT('Ctrl Pts',(-25.122293720064,-0.98553195302638,-2.83354369456912));
#5802=CARTESIAN_POINT('Ctrl Pts',(-25.1085795345898,-0.970507349552267,
-2.83872915299998));
#5803=CARTESIAN_POINT('Ctrl Pts',(-25.0817384653232,-0.9396374697407,-2.84909618968299));
#5804=CARTESIAN_POINT('Ctrl Pts',(-25.0686121956922,-0.923792524689856,
-2.85427759753642));
#5805=CARTESIAN_POINT('Ctrl Pts',(-25.0493658734545,-0.89939302142587,-2.86202163910769));
#5806=CARTESIAN_POINT('Ctrl Pts',(-25.043017487774,-0.89114441813432,-2.86460120904707));
#5807=CARTESIAN_POINT('Ctrl Pts',(-25.0305207080603,-0.874501431709215,
-2.86972568743742));
#5808=CARTESIAN_POINT('Ctrl Pts',(-25.0243713909441,-0.866107457626747,
-2.87227076450331));
#5809=CARTESIAN_POINT('Ctrl Pts',(-24.9941176023294,-0.823767677123209,
-2.88490127988302));
#5810=CARTESIAN_POINT('Ctrl Pts',(-24.97147225811,-0.788728779396106,-2.89470358965755));
#5811=CARTESIAN_POINT('Ctrl Pts',(-24.9292312229828,-0.716311799075431,
-2.9134684860099));
#5812=CARTESIAN_POINT('Ctrl Pts',(-24.9096337112948,-0.678934474646847,
-2.92243229488294));
#5813=CARTESIAN_POINT('Ctrl Pts',(-24.8825415051001,-0.621060303181762,
-2.93507687968496));
#5814=CARTESIAN_POINT('Ctrl Pts',(-24.8738954614447,-0.601467085362859,
-2.93915828390893));
#5815=CARTESIAN_POINT('Ctrl Pts',(-24.8573860335644,-0.561660534816688,
-2.94702417229759));
#5816=CARTESIAN_POINT('Ctrl Pts',(-24.8495222347111,-0.541445118061438,
-2.95080889756673));
#5817=CARTESIAN_POINT('Ctrl Pts',(-24.8383296294352,-0.510647204231348,
-2.95623934885627));
#5818=CARTESIAN_POINT('Ctrl Pts',(-24.8346943538624,-0.500285572119669,
-2.95801084324021));
#5819=CARTESIAN_POINT('Ctrl Pts',(-24.8276507980447,-0.479467813925564,
-2.96145644444383));
#5820=CARTESIAN_POINT('Ctrl Pts',(-24.8242486897808,-0.469031540585879,
-2.96312749437883));
#5821=CARTESIAN_POINT('Ctrl Pts',(-24.8143975220266,-0.437635545407871,
-2.967983313185));
#5822=CARTESIAN_POINT('Ctrl Pts',(-24.8082918810615,-0.416559413593511,
-2.97101630939715));
#5823=CARTESIAN_POINT('Ctrl Pts',(-24.79700967936,-0.374165575587155,-2.97665244169902));
#5824=CARTESIAN_POINT('Ctrl Pts',(-24.7918302021315,-0.352839925216633,
-2.97925701409689));
#5825=CARTESIAN_POINT('Ctrl Pts',(-24.782389529693,-0.309931149531079,-2.98402597733368));
#5826=CARTESIAN_POINT('Ctrl Pts',(-24.77812834015,-0.288348024079469,-2.98619038155605));
#5827=CARTESIAN_POINT('Ctrl Pts',(-24.7705262413241,-0.24492258799079,-2.99006529803462));
#5828=CARTESIAN_POINT('Ctrl Pts',(-24.767185323199,-0.223080280695769,-2.9917758240911));
#5829=CARTESIAN_POINT('Ctrl Pts',(-24.7614327168412,-0.179133051352737,
-2.99472848957151));
#5830=CARTESIAN_POINT('Ctrl Pts',(-24.7590210045444,-0.157028136357559,
-2.99597064391189));
#5831=CARTESIAN_POINT('Ctrl Pts',(-24.7551430015195,-0.112550450866729,
-2.99797103284412));
#5832=CARTESIAN_POINT('Ctrl Pts',(-24.7536770371529,-0.0901765544388105,
-2.99872909299961));
#5833=CARTESIAN_POINT('Ctrl Pts',(-24.7522040612047,-0.0564128194848313,
-2.9994911778993));
#5834=CARTESIAN_POINT('Ctrl Pts',(-24.7518343852008,-0.0451068922413159,
-2.999682558101));
#5835=CARTESIAN_POINT('Ctrl Pts',(-24.7513427166217,-0.0225174680468727,
-2.99993712712975));
#5836=CARTESIAN_POINT('Ctrl Pts',(-24.7512203639079,-0.0112452244724441,
-3.00000050164314));
#5837=CARTESIAN_POINT('Ctrl Pts',(-24.7512205732181,1.27647900817359E-15,
-3.00000039251396));
#5838=CARTESIAN_POINT('Ctrl Pts',(-24.925,9.1987778071817E-16,-2.60755260924174));
#5839=CARTESIAN_POINT('Ctrl Pts',(-24.9250003566431,0.0166541858892919,
-2.60755241953505));
#5840=CARTESIAN_POINT('Ctrl Pts',(-24.9254160783661,0.0332581559508148,
-2.60733265858178));
#5841=CARTESIAN_POINT('Ctrl Pts',(-24.9270649354643,0.0663304974791159,
-2.60646231020682));
#5842=CARTESIAN_POINT('Ctrl Pts',(-24.9282977615931,0.0828051219601012,
-2.60581189691126));
#5843=CARTESIAN_POINT('Ctrl Pts',(-24.9332076090917,0.132046707858214,-2.60322787601198));
#5844=CARTESIAN_POINT('Ctrl Pts',(-24.9380956117425,0.164639289236405,-2.60066047948669));
#5845=CARTESIAN_POINT('Ctrl Pts',(-24.9478395671871,0.213143553563254,-2.59559297392187));
#5846=CARTESIAN_POINT('Ctrl Pts',(-24.9514952030343,0.229263645988802,-2.59369843168222));
#5847=CARTESIAN_POINT('Ctrl Pts',(-24.9575851418319,0.253332291674964,-2.59055979222182));
#5848=CARTESIAN_POINT('Ctrl Pts',(-24.9597188141185,0.261344691370318,-2.58946279377858));
#5849=CARTESIAN_POINT('Ctrl Pts',(-24.9641906612921,0.2773345184445,-2.5871703966394));
#5850=CARTESIAN_POINT('Ctrl Pts',(-24.966530765891,0.28531677926617,-2.58597403111896));
#5851=CARTESIAN_POINT('Ctrl Pts',(-24.973820513222,0.309081961524918,-2.58225915775742));
#5852=CARTESIAN_POINT('Ctrl Pts',(-24.9790484377681,0.32472379379895,-2.57961022574372));
#5853=CARTESIAN_POINT('Ctrl Pts',(-24.9902256908821,0.355621851323136,-2.57399040352468));
#5854=CARTESIAN_POINT('Ctrl Pts',(-24.9961745187184,0.370877172015151,-2.57101975041035));
#5855=CARTESIAN_POINT('Ctrl Pts',(-25.0150836576248,0.416076046241271,-2.56166046299739));
#5856=CARTESIAN_POINT('Ctrl Pts',(-25.0291043543913,0.445453982261496,-2.55482429402179));
#5857=CARTESIAN_POINT('Ctrl Pts',(-25.0522383184702,0.488417442273934,-2.54380826092922));
#5858=CARTESIAN_POINT('Ctrl Pts',(-25.0603014453932,0.502555351656385,-2.54000886254706));
#5859=CARTESIAN_POINT('Ctrl Pts',(-25.0771344181921,0.530461627229326,-2.53217843551043));
#5860=CARTESIAN_POINT('Ctrl Pts',(-25.0859109306211,0.544239963564886,-2.52814434334756));
#5861=CARTESIAN_POINT('Ctrl Pts',(-25.1041597996001,0.571392063284264,-2.51987677295434));
#5862=CARTESIAN_POINT('Ctrl Pts',(-25.1135652356457,0.584667955785163,-2.51567359591457));
#5863=CARTESIAN_POINT('Ctrl Pts',(-25.1329503931644,0.610672109363501,-2.50714732573441));
#5864=CARTESIAN_POINT('Ctrl Pts',(-25.1429262744659,0.623394578020974,-2.50282595067222));
#5865=CARTESIAN_POINT('Ctrl Pts',(-25.1736949347874,0.660743188336082,-2.48973044146156));
#5866=CARTESIAN_POINT('Ctrl Pts',(-25.1953265696652,0.684552408790024,-2.4808244164163));
#5867=CARTESIAN_POINT('Ctrl Pts',(-25.2294621790932,0.718669526189459,-2.46737442476457));
#5868=CARTESIAN_POINT('Ctrl Pts',(-25.2411226141971,0.729775262858413,-2.46287588038061));
#5869=CARTESIAN_POINT('Ctrl Pts',(-25.2650163395358,0.751453108570395,-2.45387816269177));
#5870=CARTESIAN_POINT('Ctrl Pts',(-25.2772554632753,0.762029504500182,-2.44937698167526));
#5871=CARTESIAN_POINT('Ctrl Pts',(-25.3022971286317,0.782626892006878,-2.44041267983555));
#5872=CARTESIAN_POINT('Ctrl Pts',(-25.315157197433,0.792689421921388,-2.43593042229926));
#5873=CARTESIAN_POINT('Ctrl Pts',(-25.3412327555041,0.812083164942921,-2.4271128386545));
#5874=CARTESIAN_POINT('Ctrl Pts',(-25.3544672859955,0.821434074532995,-2.4227697238751));
#5875=CARTESIAN_POINT('Ctrl Pts',(-25.3813264071519,0.839452527788184,-2.41424554238548));
#5876=CARTESIAN_POINT('Ctrl Pts',(-25.3949513697869,0.848120793930839,-2.41006421940508));
#5877=CARTESIAN_POINT('Ctrl Pts',(-25.4225940554056,0.864782458141239,-2.40189271204071));
#5878=CARTESIAN_POINT('Ctrl Pts',(-25.4366117834694,0.872775835903154,-2.39790249830953));
#5879=CARTESIAN_POINT('Ctrl Pts',(-25.479261734589,0.89574572391242,-2.38626398652599));
#5880=CARTESIAN_POINT('Ctrl Pts',(-25.5084958123966,0.909716954879009,-2.37894574292179));
#5881=CARTESIAN_POINT('Ctrl Pts',(-25.5535776615725,0.928607298291761,-2.36882679203485));
#5882=CARTESIAN_POINT('Ctrl Pts',(-25.5688253899689,0.934563660377401,-2.36559439343672));
#5883=CARTESIAN_POINT('Ctrl Pts',(-25.5920023693806,0.942963605388764,-2.36098892152974));
#5884=CARTESIAN_POINT('Ctrl Pts',(-25.5997879839068,0.945677166439889,-2.35949277008248));
#5885=CARTESIAN_POINT('Ctrl Pts',(-25.6154612044866,0.950922793268217,-2.35658631440841));
#5886=CARTESIAN_POINT('Ctrl Pts',(-25.6233613960042,0.953458374961467,-2.35517402568801));
#5887=CARTESIAN_POINT('Ctrl Pts',(-25.6470876486476,0.960748669979317,-2.35109499689055));
#5888=CARTESIAN_POINT('Ctrl Pts',(-25.6629694924038,0.965199959788433,-2.34857921219018));
#5889=CARTESIAN_POINT('Ctrl Pts',(-25.6948784413748,0.97330109610864,-2.34396841563554));
#5890=CARTESIAN_POINT('Ctrl Pts',(-25.710902645268,0.976950283068507,-2.34187376666203));
#5891=CARTESIAN_POINT('Ctrl Pts',(-25.7591844222773,0.986703415822537,-2.33624500537069));
#5892=CARTESIAN_POINT('Ctrl Pts',(-25.791650783833,0.991615665333942,-2.33336629059961));
#5893=CARTESIAN_POINT('Ctrl Pts',(-25.8407756179032,0.996582697577232,-2.33044584989519));
#5894=CARTESIAN_POINT('Ctrl Pts',(-25.8572215351598,0.997837487879419,-2.32970524177098));
#5895=CARTESIAN_POINT('Ctrl Pts',(-25.8902578614934,0.999533165226665,-2.3287035410661));
#5896=CARTESIAN_POINT('Ctrl Pts',(-25.9068578724972,0.999973524878361,-2.32844279123644));
#5897=CARTESIAN_POINT('Ctrl Pts',(-25.940167362761,1.0000242628141,-2.32841276730313));
#5898=CARTESIAN_POINT('Ctrl Pts',(-25.9569704588412,0.999628762374181,-2.32864698234143));
#5899=CARTESIAN_POINT('Ctrl Pts',(-25.9903233075244,0.998003316619995,-2.32960735397221));
#5900=CARTESIAN_POINT('Ctrl Pts',(-26.0069064582144,0.99677776727011,-2.33033089082928));
#5901=CARTESIAN_POINT('Ctrl Pts',(-26.0398870987565,0.993516757651968,-2.33224874868743));
#5902=CARTESIAN_POINT('Ctrl Pts',(-26.0562852280577,0.991481744891028,-2.3334427918359));
#5903=CARTESIAN_POINT('Ctrl Pts',(-26.0889006503167,0.986614637292694,-2.3362833255874));
#5904=CARTESIAN_POINT('Ctrl Pts',(-26.1051179364934,0.983782507538744,-2.33792982096872));
#5905=CARTESIAN_POINT('Ctrl Pts',(-26.1535021710044,0.974099057442963,-2.3435209510113));
#5906=CARTESIAN_POINT('Ctrl Pts',(-26.1854056292135,0.966060458399383,-2.34811896256439));
#5907=CARTESIAN_POINT('Ctrl Pts',(-26.2248342916283,0.954027413144458,-2.35485651240158));
#5908=CARTESIAN_POINT('Ctrl Pts',(-26.2327013987641,0.951518784920254,-2.35625480890823));
#5909=CARTESIAN_POINT('Ctrl Pts',(-26.2483827345867,0.946304393522069,-2.35914625498641));
#5910=CARTESIAN_POINT('Ctrl Pts',(-26.2562117486977,0.943592705045449,-2.36064260344911));
#5911=CARTESIAN_POINT('Ctrl Pts',(-26.2795250530157,0.935192248164097,-2.36525212598659));
#5912=CARTESIAN_POINT('Ctrl Pts',(-26.2948382163531,0.929240340102425,-2.36848474521894));
#5913=CARTESIAN_POINT('Ctrl Pts',(-26.325052120344,0.916638547977858,-2.37524073173656));
#5914=CARTESIAN_POINT('Ctrl Pts',(-26.3399478665267,0.909990622039622,-2.37876303600402));
#5915=CARTESIAN_POINT('Ctrl Pts',(-26.3693289871196,0.89601139589608,-2.38606310676973));
#5916=CARTESIAN_POINT('Ctrl Pts',(-26.3838143473607,0.888680076643437,-2.38984089454832));
#5917=CARTESIAN_POINT('Ctrl Pts',(-26.4123832482896,0.873338683184519,-2.39762023550669));
#5918=CARTESIAN_POINT('Ctrl Pts',(-26.4264667819849,0.865328603021504,-2.40162180862373));
#5919=CARTESIAN_POINT('Ctrl Pts',(-26.4542373250601,0.848628527049356,-2.40981807440536));
#5920=CARTESIAN_POINT('Ctrl Pts',(-26.4679244024272,0.839938487173804,-2.41401280980997));
#5921=CARTESIAN_POINT('Ctrl Pts',(-26.4949038618745,0.821871746929689,-2.42256536268357));
#5922=CARTESIAN_POINT('Ctrl Pts',(-26.5081993038235,0.812492795486006,-2.4269242196594));
#5923=CARTESIAN_POINT('Ctrl Pts',(-26.5343829028199,0.793043775382973,-2.43577160005358));
#5924=CARTESIAN_POINT('Ctrl Pts',(-26.5471738340693,0.783046380384102,-2.44022699893485));
#5925=CARTESIAN_POINT('Ctrl Pts',(-26.5721868510483,0.762503182417989,-2.44917380576989));
#5926=CARTESIAN_POINT('Ctrl Pts',(-26.5844064334615,0.751959204775379,-2.45366439347183));
#5927=CARTESIAN_POINT('Ctrl Pts',(-26.6082843084103,0.730330096168269,-2.46264911716721));
#5928=CARTESIAN_POINT('Ctrl Pts',(-26.6199425628188,0.719244941847823,-2.46714330180597));
#5929=CARTESIAN_POINT('Ctrl Pts',(-26.6540867150583,0.685176365586002,-2.4805866593511));
#5930=CARTESIAN_POINT('Ctrl Pts',(-26.6757462073237,0.661378975879614,-2.48949782346476));
#5931=CARTESIAN_POINT('Ctrl Pts',(-26.706573146655,0.624022706324936,-2.50261037529356));
#5932=CARTESIAN_POINT('Ctrl Pts',(-26.7165759724886,0.611286384102533,-2.50694112711596));
#5933=CARTESIAN_POINT('Ctrl Pts',(-26.7311533876529,0.591762476370502,-2.51334967146032));
#5934=CARTESIAN_POINT('Ctrl Pts',(-26.7359451890069,0.585178854079478,-2.51547299658856));
#5935=CARTESIAN_POINT('Ctrl Pts',(-26.7453814833122,0.571874856074331,-2.51968511284942));
#5936=CARTESIAN_POINT('Ctrl Pts',(-26.7500351366602,0.565140645160058,-2.52177806865427));
#5937=CARTESIAN_POINT('Ctrl Pts',(-26.7637222516845,0.544804309725441,-2.52797665659195));
#5938=CARTESIAN_POINT('Ctrl Pts',(-26.7724803391795,0.531075645530331,-2.53200078580807));
#5939=CARTESIAN_POINT('Ctrl Pts',(-26.7892946991393,0.503248393728805,-2.53981950802604));
#5940=CARTESIAN_POINT('Ctrl Pts',(-26.7973477617837,0.489154779345304,-2.54361267297452));
#5941=CARTESIAN_POINT('Ctrl Pts',(-26.8204545728126,0.446333368005566,-2.55461135090606));
#5942=CARTESIAN_POINT('Ctrl Pts',(-26.834458477791,0.417066232433272,-2.56143651401678));
#5943=CARTESIAN_POINT('Ctrl Pts',(-26.8596488370896,0.357057925052848,-2.57389950485306));
#5944=CARTESIAN_POINT('Ctrl Pts',(-26.8708365853539,0.326307436876508,-2.57953848796631));
#5945=CARTESIAN_POINT('Ctrl Pts',(-26.8854203844307,0.279045599412755,-2.58696737317912));
#5946=CARTESIAN_POINT('Ctrl Pts',(-26.8899176876621,0.263080836121059,-2.5892735666817));
#5947=CARTESIAN_POINT('Ctrl Pts',(-26.8981471118759,0.230786385702432,-2.59351339304776));
#5948=CARTESIAN_POINT('Ctrl Pts',(-26.901854302142,0.21455390787461,-2.59543412523401));
#5949=CARTESIAN_POINT('Ctrl Pts',(-26.9084607843892,0.18188620301005,-2.59886924230701));
#5950=CARTESIAN_POINT('Ctrl Pts',(-26.9113574905324,0.165464138876775,-2.60038228698979));
#5951=CARTESIAN_POINT('Ctrl Pts',(-26.9163383589761,0.132393422445161,-2.60299055921657));
#5952=CARTESIAN_POINT('Ctrl Pts',(-26.9184105531932,0.115817718038398,-2.60407951595308));
#5953=CARTESIAN_POINT('Ctrl Pts',(-26.9233593618272,0.0661859402484169,
-2.60668400705037));
#5954=CARTESIAN_POINT('Ctrl Pts',(-26.9249972922528,0.0331164849794912,
-2.60755116529973));
#5955=CARTESIAN_POINT('Ctrl Pts',(-26.9250013487368,-0.0164341042586774,
-2.60755332849862));
#5956=CARTESIAN_POINT('Ctrl Pts',(-26.924593771391,-0.0329435135702297,
-2.60733786318111));
#5957=CARTESIAN_POINT('Ctrl Pts',(-26.9229598784543,-0.0659474161951027,
-2.60647540292583));
#5958=CARTESIAN_POINT('Ctrl Pts',(-26.9217335860717,-0.0824419098590701,
-2.60582840846347));
#5959=CARTESIAN_POINT('Ctrl Pts',(-26.9184554239328,-0.115415878608659,
-2.60410310617676));
#5960=CARTESIAN_POINT('Ctrl Pts',(-26.9164025400161,-0.13189883452203,-2.60302426431672));
#5961=CARTESIAN_POINT('Ctrl Pts',(-26.9114621352338,-0.164835602978563,
-2.60043699179504));
#5962=CARTESIAN_POINT('Ctrl Pts',(-26.9085613270678,-0.181339949722123,
-2.59892168747798));
#5963=CARTESIAN_POINT('Ctrl Pts',(-26.9019944221297,-0.213908268855235,
-2.59550682162745));
#5964=CARTESIAN_POINT('Ctrl Pts',(-26.8983181557808,-0.230051496944324,
-2.59360192011071));
#5965=CARTESIAN_POINT('Ctrl Pts',(-26.8902038146127,-0.262018183387908,
-2.58942059752268));
#5966=CARTESIAN_POINT('Ctrl Pts',(-26.8857646886985,-0.277849358655751,
-2.58714361859993));
#5967=CARTESIAN_POINT('Ctrl Pts',(-26.8713188216695,-0.324895801813619,
-2.57978251945632));
#5968=CARTESIAN_POINT('Ctrl Pts',(-26.8601834035885,-0.355670011650629,
-2.57416690219528));
#5969=CARTESIAN_POINT('Ctrl Pts',(-26.8412500664846,-0.400941255234936,
-2.56479529641425));
#5970=CARTESIAN_POINT('Ctrl Pts',(-26.8345604461981,-0.415894450482954,
-2.56151035689195));
#5971=CARTESIAN_POINT('Ctrl Pts',(-26.8239684235737,-0.43809039102524,-2.55636178150266));
#5972=CARTESIAN_POINT('Ctrl Pts',(-26.8203410661095,-0.445456832661156,
-2.55460695983524));
#5973=CARTESIAN_POINT('Ctrl Pts',(-26.8128999456829,-0.460110113434816,
-2.55102621846156));
#5974=CARTESIAN_POINT('Ctrl Pts',(-26.8090809400854,-0.467406099051344,
-2.54919783195028));
#5975=CARTESIAN_POINT('Ctrl Pts',(-26.7973956024953,-0.489075501379373,
-2.54363495988491));
#5976=CARTESIAN_POINT('Ctrl Pts',(-26.7892904087949,-0.503256366320303,
-2.53981745826163));
#5977=CARTESIAN_POINT('Ctrl Pts',(-26.7724556899274,-0.531115565582874,
-2.53198937867127));
#5978=CARTESIAN_POINT('Ctrl Pts',(-26.7637274203706,-0.544791910987859,
-2.52797935716389));
#5979=CARTESIAN_POINT('Ctrl Pts',(-26.7366217266702,-0.58507967901889,-2.51570272134658));
#5980=CARTESIAN_POINT('Ctrl Pts',(-26.7173257403855,-0.610951467196291,
-2.5071891514559));
#5981=CARTESIAN_POINT('Ctrl Pts',(-26.6865421652591,-0.648316199104958,
-2.49408756309349));
#5982=CARTESIAN_POINT('Ctrl Pts',(-26.6759737885839,-0.660530164014686,
-2.4896650790417));
#5983=CARTESIAN_POINT('Ctrl Pts',(-26.6542143618837,-0.68447654199776,-2.48073725881265));
#5984=CARTESIAN_POINT('Ctrl Pts',(-26.6430275831957,-0.696204572944766,
-2.47623358134868));
#5985=CARTESIAN_POINT('Ctrl Pts',(-26.625757459411,-0.713446061713053,-2.46943219638784));
#5986=CARTESIAN_POINT('Ctrl Pts',(-26.619921440287,-0.71913160109651,-2.46715852858782));
#5987=CARTESIAN_POINT('Ctrl Pts',(-26.6081492806517,-0.730323844266243,
-2.46262464724449));
#5988=CARTESIAN_POINT('Ctrl Pts',(-26.6022023493564,-0.735841448132365,
-2.4603601639289));
#5989=CARTESIAN_POINT('Ctrl Pts',(-26.5841990801845,-0.752142596351643,
-2.45358727585739));
#5990=CARTESIAN_POINT('Ctrl Pts',(-26.5719637153137,-0.762691293347727,
-2.44909283533732));
#5991=CARTESIAN_POINT('Ctrl Pts',(-26.5345859666616,-0.793375000104388,
-2.43572683396233));
#5992=CARTESIAN_POINT('Ctrl Pts',(-26.5087543078564,-0.812569281368951,
-2.42696429363964));
#5993=CARTESIAN_POINT('Ctrl Pts',(-26.4686216279805,-0.839484914822932,
-2.41422981442001));
#5994=CARTESIAN_POINT('Ctrl Pts',(-26.4550122677061,-0.848144060795981,
-2.41005301554825));
#5995=CARTESIAN_POINT('Ctrl Pts',(-26.4273198206187,-0.864833014186361,
-2.40186770943339));
#5996=CARTESIAN_POINT('Ctrl Pts',(-26.4132367723247,-0.872862861793055,
-2.39785915569382));
#5997=CARTESIAN_POINT('Ctrl Pts',(-26.3845827730249,-0.888283954759515,
-2.39004399122573));
#5998=CARTESIAN_POINT('Ctrl Pts',(-26.3700175910458,-0.895672296665481,
-2.38623887159212));
#5999=CARTESIAN_POINT('Ctrl Pts',(-26.3477725177819,-0.906273162875092,
-2.38070494715482));
#6000=CARTESIAN_POINT('Ctrl Pts',(-26.3402926727503,-0.909725000544915,
-2.37888997766033));
#6001=CARTESIAN_POINT('Ctrl Pts',(-26.3252947580114,-0.916423170547351,
-2.37534522135331));
#6002=CARTESIAN_POINT('Ctrl Pts',(-26.3177609641362,-0.919677618978278,
-2.37361127867653));
#6003=CARTESIAN_POINT('Ctrl Pts',(-26.279960326246,-0.935453358182183,-2.36515451304931));
#6004=CARTESIAN_POINT('Ctrl Pts',(-26.2492308175849,-0.946541064909447,
-2.35904578187963));
#6005=CARTESIAN_POINT('Ctrl Pts',(-26.1868089918217,-0.96567161724459,-2.34833908445429));
#6006=CARTESIAN_POINT('Ctrl Pts',(-26.1551127594127,-0.973718288717797,
-2.34373917694448));
#6007=CARTESIAN_POINT('Ctrl Pts',(-26.1068144462703,-0.983469972772359,
-2.33811102541251));
#6008=CARTESIAN_POINT('Ctrl Pts',(-26.090589178399,-0.986333510705604,-2.33644692696739));
#6009=CARTESIAN_POINT('Ctrl Pts',(-26.0578800212193,-0.991270124222091,
-2.33356672209884));
#6010=CARTESIAN_POINT('Ctrl Pts',(-26.0413989600866,-0.993342685095569,
-2.33235094950618));
#6011=CARTESIAN_POINT('Ctrl Pts',(-26.016468400417,-0.995843155056376,-2.33088062949275));
#6012=CARTESIAN_POINT('Ctrl Pts',(-26.0081137802036,-0.996575200948386,
-2.33044941555121));
#6013=CARTESIAN_POINT('Ctrl Pts',(-25.9914406456729,-0.997825328960477,
-2.32971229361946));
#6014=CARTESIAN_POINT('Ctrl Pts',(-25.9831090698346,-0.998345104091185,
-2.32940539355605));
#6015=CARTESIAN_POINT('Ctrl Pts',(-25.9581619918789,-0.999588413090816,
-2.32867085845433));
#6016=CARTESIAN_POINT('Ctrl Pts',(-25.9415535789236,-1.00000042873077,-2.32842685045339));
#6017=CARTESIAN_POINT('Ctrl Pts',(-25.8918801116584,-0.999999142511445,
-2.3284276733473));
#6018=CARTESIAN_POINT('Ctrl Pts',(-25.8588976369251,-0.998358102087351,
-2.32940162628821));
#6019=CARTESIAN_POINT('Ctrl Pts',(-25.809655452566,-0.993462469088689,-2.33228059590286));
#6020=CARTESIAN_POINT('Ctrl Pts',(-25.7932780679245,-0.991424398396009,
-2.3334763859153));
#6021=CARTESIAN_POINT('Ctrl Pts',(-25.7605967018549,-0.986531578876193,
-2.3363316707559));
#6022=CARTESIAN_POINT('Ctrl Pts',(-25.744287250752,-0.983675445441527,-2.33799197788889));
#6023=CARTESIAN_POINT('Ctrl Pts',(-25.7198948761487,-0.978775245710681,
-2.34082078278937));
#6024=CARTESIAN_POINT('Ctrl Pts',(-25.7117693154796,-0.97703729202741,-2.34182114664375));
#6025=CARTESIAN_POINT('Ctrl Pts',(-25.6955363910876,-0.973352864470024,
-2.34393407887513));
#6026=CARTESIAN_POINT('Ctrl Pts',(-25.6874340994824,-0.971407041360755,
-2.34504624803507));
#6027=CARTESIAN_POINT('Ctrl Pts',(-25.6632984183101,-0.965291239666667,
-2.34852759864218));
#6028=CARTESIAN_POINT('Ctrl Pts',(-25.6473893995262,-0.960834612092797,
-2.35104651772393));
#6029=CARTESIAN_POINT('Ctrl Pts',(-25.6159251530686,-0.951180080790836,
-2.35644914953995));
#6030=CARTESIAN_POINT('Ctrl Pts',(-25.6003693864664,-0.945982332371019,
-2.35933277792));
#6031=CARTESIAN_POINT('Ctrl Pts',(-25.5696010487147,-0.934857849827407,
-2.36543410266167));
#6032=CARTESIAN_POINT('Ctrl Pts',(-25.554388497757,-0.928931075544406,-2.36865182569907));
#6033=CARTESIAN_POINT('Ctrl Pts',(-25.5092553225566,-0.910065915709693,
-2.37876175430699));
#6034=CARTESIAN_POINT('Ctrl Pts',(-25.4798364380125,-0.896042727572783,
-2.38611169599139));
#6035=CARTESIAN_POINT('Ctrl Pts',(-25.4438909156586,-0.876699211680765,
-2.39591502278521));
#6036=CARTESIAN_POINT('Ctrl Pts',(-25.4367414461902,-0.872737300160875,
-2.39790741951297));
#6037=CARTESIAN_POINT('Ctrl Pts',(-25.4225293356803,-0.864633016249675,
-2.4019490228773));
#6038=CARTESIAN_POINT('Ctrl Pts',(-25.4154580969326,-0.860484766397168,
-2.40400099723934));
#6039=CARTESIAN_POINT('Ctrl Pts',(-25.3944657161042,-0.847820800232132,
-2.41021024122676));
#6040=CARTESIAN_POINT('Ctrl Pts',(-25.380746070164,-0.839077244133132,-2.41442548123447));
#6041=CARTESIAN_POINT('Ctrl Pts',(-25.3538260232817,-0.820989195886628,
-2.42297767676367));
#6042=CARTESIAN_POINT('Ctrl Pts',(-25.3406279393829,-0.811646297981063,
-2.42731389565942));
#6043=CARTESIAN_POINT('Ctrl Pts',(-25.3147430597672,-0.792367900936232,
-2.4360740734985));
#6044=CARTESIAN_POINT('Ctrl Pts',(-25.3020562810124,-0.782432389835531,
-2.44049806007426));
#6045=CARTESIAN_POINT('Ctrl Pts',(-25.2771860341754,-0.761968758341592,
-2.44940268163808));
#6046=CARTESIAN_POINT('Ctrl Pts',(-25.2650025732109,-0.751440637442869,
-2.45388334271683));
#6047=CARTESIAN_POINT('Ctrl Pts',(-25.2411353303519,-0.729786781206716,
-2.46287109582097));
#6048=CARTESIAN_POINT('Ctrl Pts',(-25.2294515461917,-0.718661056693565,
-2.46737821378511));
#6049=CARTESIAN_POINT('Ctrl Pts',(-25.2065843288473,-0.695801899103858,
-2.47638907712377));
#6050=CARTESIAN_POINT('Ctrl Pts',(-25.1954014188971,-0.684068711345196,
-2.48089267439044));
#6051=CARTESIAN_POINT('Ctrl Pts',(-25.1790045373378,-0.666000870018047,
-2.48762367211152));
#6052=CARTESIAN_POINT('Ctrl Pts',(-25.1735960376354,-0.659892776183962,
-2.48986579326022));
#6053=CARTESIAN_POINT('Ctrl Pts',(-25.1629494208789,-0.647568638488022,
-2.49431990834337));
#6054=CARTESIAN_POINT('Ctrl Pts',(-25.1577105174054,-0.641352897528938,
-2.49653204883514));
#6055=CARTESIAN_POINT('Ctrl Pts',(-25.1319358378313,-0.610000274169448,
-2.50751029184405));
#6056=CARTESIAN_POINT('Ctrl Pts',(-25.1126431635002,-0.584053957250262,
-2.51603030353833));
#6057=CARTESIAN_POINT('Ctrl Pts',(-25.0766559633797,-0.530429156133724,
-2.5323404528869));
#6058=CARTESIAN_POINT('Ctrl Pts',(-25.0599598863832,-0.5027512333643,-2.54013165293878));
#6059=CARTESIAN_POINT('Ctrl Pts',(-25.0368787132278,-0.459895387665408,
-2.55112212486567));
#6060=CARTESIAN_POINT('Ctrl Pts',(-25.0295127265205,-0.445386602515357,
-2.55466961647923));
#6061=CARTESIAN_POINT('Ctrl Pts',(-25.015447538885,-0.415909836891661,-2.56150652151534));
#6062=CARTESIAN_POINT('Ctrl Pts',(-25.0087479847154,-0.400940313195677,
-2.56479614450174));
#6063=CARTESIAN_POINT('Ctrl Pts',(-24.9992124578344,-0.378134446441367,
-2.56951620636083));
#6064=CARTESIAN_POINT('Ctrl Pts',(-24.9961153890925,-0.370461653972982,
-2.57105596109367));
#6065=CARTESIAN_POINT('Ctrl Pts',(-24.9901146400105,-0.355046096214791,
-2.57405082283813));
#6066=CARTESIAN_POINT('Ctrl Pts',(-24.9872162178828,-0.347318031889453,
-2.57550327285404));
#6067=CARTESIAN_POINT('Ctrl Pts',(-24.978823527118,-0.324069285671267,-2.57972387330155));
#6068=CARTESIAN_POINT('Ctrl Pts',(-24.9736218334904,-0.308462402151713,
-2.58236010535197));
#6069=CARTESIAN_POINT('Ctrl Pts',(-24.9640099750406,-0.277069749192375,
-2.58725894187428));
#6070=CARTESIAN_POINT('Ctrl Pts',(-24.9595973255169,-0.261278097086916,
-2.58952279476208));
#6071=CARTESIAN_POINT('Ctrl Pts',(-24.9515543557535,-0.229504132582814,
-2.59366790173024));
#6072=CARTESIAN_POINT('Ctrl Pts',(-24.9479240403419,-0.213521820083151,
-2.59554916744326));
#6073=CARTESIAN_POINT('Ctrl Pts',(-24.941447441202,-0.181365268356563,-2.59891718319403));
#6074=CARTESIAN_POINT('Ctrl Pts',(-24.9386011499407,-0.165191031604557,
-2.60040394522676));
#6075=CARTESIAN_POINT('Ctrl Pts',(-24.9337002237304,-0.132648091777223,
-2.60297035508352));
#6076=CARTESIAN_POINT('Ctrl Pts',(-24.93164556828,-0.116279393924668,-2.60405001587271));
#6077=CARTESIAN_POINT('Ctrl Pts',(-24.928341708171,-0.0833436511207354,
-2.60578872210514));
#6078=CARTESIAN_POINT('Ctrl Pts',(-24.9270927815557,-0.0667757724171859,
-2.60644761593104));
#6079=CARTESIAN_POINT('Ctrl Pts',(-24.9258378814317,-0.0417737140066712,
-2.60711000800062));
#6080=CARTESIAN_POINT('Ctrl Pts',(-24.9255229363957,-0.0334016706388513,
-2.60727635262695));
#6081=CARTESIAN_POINT('Ctrl Pts',(-24.9251040599288,-0.016674193542247,
-2.60749761997638));
#6082=CARTESIAN_POINT('Ctrl Pts',(-24.9249998216785,-0.00832709294464443,
-2.60755270409509));
#6083=CARTESIAN_POINT('Ctrl Pts',(-24.925,9.1987778071817E-16,-2.60755260924174));
#6084=CARTESIAN_POINT('',(-27.0987792489536,0.000111760644532478,-2.99999999791826));
#6085=CARTESIAN_POINT('',(-24.7512207470268,1.19503331376525E-15,-3.));
#6086=CARTESIAN_POINT('Ctrl Pts',(-27.0987792482096,0.000121760644497039,
-2.99999999752906));
#6087=CARTESIAN_POINT('Ctrl Pts',(-27.098788174959,-0.125283846590266,-3.00000466933289));
#6088=CARTESIAN_POINT('Ctrl Pts',(-27.0836572608919,-0.249887612487901,
-2.99204806120949));
#6089=CARTESIAN_POINT('Ctrl Pts',(-27.0242841101371,-0.489247948794867,
-2.96225146824176));
#6090=CARTESIAN_POINT('Ctrl Pts',(-26.9807678619009,-0.603149705373672,
-2.94076784698443));
#6091=CARTESIAN_POINT('Ctrl Pts',(-26.8427192011915,-0.860536585811288,
-2.87814965124282));
#6092=CARTESIAN_POINT('Ctrl Pts',(-26.7376907200788,-0.989566183854094,
-2.83419679721259));
#6093=CARTESIAN_POINT('Ctrl Pts',(-26.515546731998,-1.17588715226963,-2.76143949975895));
#6094=CARTESIAN_POINT('Ctrl Pts',(-26.4004065512224,-1.24404280001843,-2.73036038773096));
#6095=CARTESIAN_POINT('Ctrl Pts',(-26.1626806024214,-1.32927584783709,-2.68979319984398));
#6096=CARTESIAN_POINT('Ctrl Pts',(-26.0452468272229,-1.35044153732407,-2.6788631272028));
#6097=CARTESIAN_POINT('Ctrl Pts',(-25.8046235970334,-1.35043417397338,-2.67886683912841));
#6098=CARTESIAN_POINT('Ctrl Pts',(-25.6870707985623,-1.32923939483633,-2.68981328055134));
#6099=CARTESIAN_POINT('Ctrl Pts',(-25.4498537631474,-1.24407674422506,-2.73034115324496));
#6100=CARTESIAN_POINT('Ctrl Pts',(-25.3353287651251,-1.17639337787322,-2.76120614485257));
#6101=CARTESIAN_POINT('Ctrl Pts',(-25.1094606312527,-0.987455834848597,
-2.83506483214697));
#6102=CARTESIAN_POINT('Ctrl Pts',(-25.0061794065515,-0.857630793523992,
-2.87869860737191));
#6103=CARTESIAN_POINT('Ctrl Pts',(-24.8702787932849,-0.60571251075133,-2.94025713869714));
#6104=CARTESIAN_POINT('Ctrl Pts',(-24.826322397393,-0.491220877835279,-2.9619507002191));
#6105=CARTESIAN_POINT('Ctrl Pts',(-24.7664326588164,-0.250724694261063,
-2.9919992973031));
#6106=CARTESIAN_POINT('Ctrl Pts',(-24.7512189476652,-0.125688720919347,
-3.));
#6107=CARTESIAN_POINT('Ctrl Pts',(-24.7512207470268,1.27935820677023E-15,
-3.));
#6108=CARTESIAN_POINT('',(-26.9249999965755,8.27588207122033E-5,-2.60755260743232));
#6109=CARTESIAN_POINT('',(-27.0987792489536,0.000111760644532478,-2.99999999791826));
#6110=CARTESIAN_POINT('',(-26.925,-1.22464679914735E-16,-2.60755336253157));
#6111=CARTESIAN_POINT('Ctrl Pts',(-26.9249999965755,8.27588207122235E-5,
-2.60755260743232));
#6112=CARTESIAN_POINT('Ctrl Pts',(-26.9249999988585,5.51724988956825E-5,
-2.6075526086923));
#6113=CARTESIAN_POINT('Ctrl Pts',(-26.925,2.75862252984736E-5,-2.60755260934744));
#6114=CARTESIAN_POINT('Ctrl Pts',(-26.925,3.70771735314531E-16,-2.60755260939776));
#6115=CARTESIAN_POINT('',(-24.925,2.76064321768413E-16,-2.60755260924174));
#6116=CARTESIAN_POINT('Ctrl Pts',(-26.925,3.70771735314531E-16,-2.60755260939776));
#6117=CARTESIAN_POINT('Ctrl Pts',(-26.925,-0.0568048545755076,-2.60755271302726));
#6118=CARTESIAN_POINT('Ctrl Pts',(-26.9201545072348,-0.11340491023354,-2.60497728285413));
#6119=CARTESIAN_POINT('Ctrl Pts',(-26.9010104955459,-0.224986239203301,
-2.5949812948901));
#6120=CARTESIAN_POINT('Ctrl Pts',(-26.8867435237432,-0.279664869028174,
-2.58757303140778));
#6121=CARTESIAN_POINT('Ctrl Pts',(-26.8304379456036,-0.439261093144541,
-2.55919607531667));
#6122=CARTESIAN_POINT('Ctrl Pts',(-26.7755419497675,-0.537393100961328,
-2.53230699136511));
#6123=CARTESIAN_POINT('Ctrl Pts',(-26.6644533472358,-0.676591305065243,
-2.48451442941931));
#6124=CARTESIAN_POINT('Ctrl Pts',(-26.6171007671406,-0.724942488787085,
-2.46539574358496));
#6125=CARTESIAN_POINT('Ctrl Pts',(-26.4737133682738,-0.844473887402714,
-2.41369606443497));
#6126=CARTESIAN_POINT('Ctrl Pts',(-26.3682038617099,-0.904656958254231,
-2.3821133442928));
#6127=CARTESIAN_POINT('Ctrl Pts',(-26.1484453864063,-0.980999063110181,
-2.34001084161919));
#6128=CARTESIAN_POINT('Ctrl Pts',(-26.0378922085562,-1.00000218800714,-2.32842180399995));
#6129=CARTESIAN_POINT('Ctrl Pts',(-25.8119011916326,-0.999997808364594,
-2.3284324547047));
#6130=CARTESIAN_POINT('Ctrl Pts',(-25.701190289908,-0.980940359915226,-2.34004920952815));
#6131=CARTESIAN_POINT('Ctrl Pts',(-25.4813838789151,-0.904439026472573,
-2.38222657916128));
#6132=CARTESIAN_POINT('Ctrl Pts',(-25.3760142250185,-0.844278486742652,
-2.41378709535207));
#6133=CARTESIAN_POINT('Ctrl Pts',(-25.1812462928252,-0.681847452255133,
-2.48402790420274));
#6134=CARTESIAN_POINT('Ctrl Pts',(-25.0955604560339,-0.575048470588128,
-2.52290226852301));
#6135=CARTESIAN_POINT('Ctrl Pts',(-24.998457233114,-0.384117255242603,-2.56961701508285));
#6136=CARTESIAN_POINT('Ctrl Pts',(-24.9711794271723,-0.310565523100878,
-2.5835333593029));
#6137=CARTESIAN_POINT('Ctrl Pts',(-24.9343517093786,-0.157452571641774,
-2.60255728285361));
#6138=CARTESIAN_POINT('Ctrl Pts',(-24.925,-0.0790612261689355,-2.6075496863545));
#6139=CARTESIAN_POINT('Ctrl Pts',(-24.925,9.22656048785168E-16,-2.60755260924175));
#6140=CARTESIAN_POINT('',(-24.7512207470268,1.19503331376525E-15,-3.));
#6141=CARTESIAN_POINT('Ctrl Pts',(-24.7512205732181,-1.76183185122132E-16,
3.00000039251396));
#6142=CARTESIAN_POINT('Ctrl Pts',(-24.7512209918384,-0.0224904489448875,
3.0000001742556));
#6143=CARTESIAN_POINT('Ctrl Pts',(-24.7517089574441,-0.0449130845232464,
2.99974733834206));
#6144=CARTESIAN_POINT('Ctrl Pts',(-24.7536443519837,-0.0895752381506375,
2.99874599882652));
#6145=CARTESIAN_POINT('Ctrl Pts',(-24.7550914179306,-0.111823200513362,
2.9979976955573));
#6146=CARTESIAN_POINT('Ctrl Pts',(-24.7608544959128,-0.178320919528189,
2.99502476849759));
#6147=CARTESIAN_POINT('Ctrl Pts',(-24.766591932863,-0.222335186723983,2.99207096785045));
#6148=CARTESIAN_POINT('Ctrl Pts',(-24.7780291872986,-0.287837198516676,
2.98624078109657));
#6149=CARTESIAN_POINT('Ctrl Pts',(-24.7823200974485,-0.30960638724731,2.98406110217344));
#6150=CARTESIAN_POINT('Ctrl Pts',(-24.789468342319,-0.342109605994453,2.98045008409494));
#6151=CARTESIAN_POINT('Ctrl Pts',(-24.7919728029526,-0.352929856681446,
2.97918798270959));
#6152=CARTESIAN_POINT('Ctrl Pts',(-24.7972217651647,-0.37452313010145,2.97655057002885));
#6153=CARTESIAN_POINT('Ctrl Pts',(-24.7999685317995,-0.385302680101395,
2.97517414639763));
#6154=CARTESIAN_POINT('Ctrl Pts',(-24.8085250872429,-0.41739609024285,2.97090016875934));
#6155=CARTESIAN_POINT('Ctrl Pts',(-24.81466151752,-0.438519418189051,2.96785256118554));
#6156=CARTESIAN_POINT('Ctrl Pts',(-24.8277811472732,-0.480245335622268,
2.96138693176614));
#6157=CARTESIAN_POINT('Ctrl Pts',(-24.8347637590013,-0.500846703560905,
2.95796918269451));
#6158=CARTESIAN_POINT('Ctrl Pts',(-24.8569589172265,-0.561884990270968,
2.94720128262928));
#6159=CARTESIAN_POINT('Ctrl Pts',(-24.8734161226417,-0.601558077547717,
2.93933624108072));
#6160=CARTESIAN_POINT('Ctrl Pts',(-24.9005702937365,-0.65957757549401,2.92666224804854));
#6161=CARTESIAN_POINT('Ctrl Pts',(-24.9100346262345,-0.678669948505794,
2.9222910240135));
#6162=CARTESIAN_POINT('Ctrl Pts',(-24.9297928233973,-0.716355649282141,
2.91328208432799));
#6163=CARTESIAN_POINT('Ctrl Pts',(-24.9400945131254,-0.734962441112178,
2.90864084409791));
#6164=CARTESIAN_POINT('Ctrl Pts',(-24.961514660095,-0.77162967400038,2.89912896911718));
#6165=CARTESIAN_POINT('Ctrl Pts',(-24.9725545674253,-0.789557946478675,
2.89429319601545));
#6166=CARTESIAN_POINT('Ctrl Pts',(-24.9953084665056,-0.824674949037347,
2.88448368582705));
#6167=CARTESIAN_POINT('Ctrl Pts',(-25.0070179507415,-0.841855856812551,
2.87951192539658));
#6168=CARTESIAN_POINT('Ctrl Pts',(-25.043133571216,-0.892292847196549,2.86444548622589));
#6169=CARTESIAN_POINT('Ctrl Pts',(-25.0685243392037,-0.924445728200638,
2.85419906644615));
#6170=CARTESIAN_POINT('Ctrl Pts',(-25.1085920152708,-0.970518787083053,
2.83872479371573));
#6171=CARTESIAN_POINT('Ctrl Pts',(-25.1222787941031,-0.985516398208712,
2.83354919922538));
#6172=CARTESIAN_POINT('Ctrl Pts',(-25.1503247573348,-1.01479098932509,2.82319728666854));
#6173=CARTESIAN_POINT('Ctrl Pts',(-25.164690788982,-1.02907375849125,2.81801865872127));
#6174=CARTESIAN_POINT('Ctrl Pts',(-25.1940841805899,-1.05688925756544,2.80770519124119));
#6175=CARTESIAN_POINT('Ctrl Pts',(-25.2091790647757,-1.07047808243068,2.80254833483866));
#6176=CARTESIAN_POINT('Ctrl Pts',(-25.2397860183817,-1.09666813400313,2.79240366726727));
#6177=CARTESIAN_POINT('Ctrl Pts',(-25.2553204379955,-1.1092959595929,2.78740689519965));
#6178=CARTESIAN_POINT('Ctrl Pts',(-25.2868471218303,-1.13362876731755,2.7775997880586));
#6179=CARTESIAN_POINT('Ctrl Pts',(-25.3028398226619,-1.1453347251136,2.77278915814535));
#6180=CARTESIAN_POINT('Ctrl Pts',(-25.3352862383422,-1.16783527307201,2.7633878040888));
#6181=CARTESIAN_POINT('Ctrl Pts',(-25.351739959153,-1.17862983581216,2.75879704618161));
#6182=CARTESIAN_POINT('Ctrl Pts',(-25.4018015943325,-1.20964925021433,2.74540688876099));
#6183=CARTESIAN_POINT('Ctrl Pts',(-25.4361159534219,-1.22851653432304,2.73698721829838));
#6184=CARTESIAN_POINT('Ctrl Pts',(-25.4890321005069,-1.2540267758302,2.72534532216722));
#6185=CARTESIAN_POINT('Ctrl Pts',(-25.5069295704027,-1.26207047477092,2.72162643380116));
#6186=CARTESIAN_POINT('Ctrl Pts',(-25.5341342320122,-1.2734140814595,2.71632781873948));
#6187=CARTESIAN_POINT('Ctrl Pts',(-25.5432728261675,-1.27707857798256,2.71460649012168));
#6188=CARTESIAN_POINT('Ctrl Pts',(-25.5616697300355,-1.2841624728764,2.71126260047887));
#6189=CARTESIAN_POINT('Ctrl Pts',(-25.5709428123064,-1.28758661927441,2.70963775628573));
#6190=CARTESIAN_POINT('Ctrl Pts',(-25.5987921995341,-1.29743171221407,2.7049448162659));
#6191=CARTESIAN_POINT('Ctrl Pts',(-25.6174339809943,-1.3034429040471,2.70205039524382));
#6192=CARTESIAN_POINT('Ctrl Pts',(-25.6548880488268,-1.31438298806204,2.69674565415259));
#6193=CARTESIAN_POINT('Ctrl Pts',(-25.6736969296858,-1.31931098956042,2.69433575157958));
#6194=CARTESIAN_POINT('Ctrl Pts',(-25.7303690862317,-1.33248199267997,2.68785983771893));
#6195=CARTESIAN_POINT('Ctrl Pts',(-25.7684774334826,-1.33911568210638,2.68454786410377));
#6196=CARTESIAN_POINT('Ctrl Pts',(-25.8261391530629,-1.34582335222856,2.6811878846237));
#6197=CARTESIAN_POINT('Ctrl Pts',(-25.8454430323917,-1.34751786899546,2.6803358118198));
#6198=CARTESIAN_POINT('Ctrl Pts',(-25.8842203925786,-1.34980777647361,2.67918335088873));
#6199=CARTESIAN_POINT('Ctrl Pts',(-25.903705143976,-1.35040245497255,2.67888335709825));
#6200=CARTESIAN_POINT('Ctrl Pts',(-25.9428031383705,-1.3504709734195,2.67884881443484));
#6201=CARTESIAN_POINT('Ctrl Pts',(-25.9625262668505,-1.34993687451433,2.67911827983488));
#6202=CARTESIAN_POINT('Ctrl Pts',(-26.0016751544636,-1.34774181046254,2.68022319148998));
#6203=CARTESIAN_POINT('Ctrl Pts',(-26.0211401155725,-1.34608678179488,2.68105562372842));
#6204=CARTESIAN_POINT('Ctrl Pts',(-26.059852112923,-1.34168298980989,2.68326212736971));
#6205=CARTESIAN_POINT('Ctrl Pts',(-26.0790998997345,-1.3389348308238,2.68463587910206));
#6206=CARTESIAN_POINT('Ctrl Pts',(-26.1173832113779,-1.3323621027606,2.6879039252919));
#6207=CARTESIAN_POINT('Ctrl Pts',(-26.1364187282489,-1.32853748653121,2.68979822524671));
#6208=CARTESIAN_POINT('Ctrl Pts',(-26.1932111473027,-1.31546058553577,2.69623084419525));
#6209=CARTESIAN_POINT('Ctrl Pts',(-26.2306587701737,-1.30460495425468,2.70152087608487));
#6210=CARTESIAN_POINT('Ctrl Pts',(-26.2769393229609,-1.28835507017719,2.70927245589678));
#6211=CARTESIAN_POINT('Ctrl Pts',(-26.2861735714613,-1.28496732277493,2.7108812019877));
#6212=CARTESIAN_POINT('Ctrl Pts',(-26.3045800008344,-1.27792560939944,2.71420782302654));
#6213=CARTESIAN_POINT('Ctrl Pts',(-26.3137695365298,-1.27426364167247,2.71592937831153));
#6214=CARTESIAN_POINT('Ctrl Pts',(-26.3411342135086,-1.26291934373526,2.72123265364054));
#6215=CARTESIAN_POINT('Ctrl Pts',(-26.359108489593,-1.25488165967842,2.72495179584752));
#6216=CARTESIAN_POINT('Ctrl Pts',(-26.3945729485003,-1.23786371810422,2.73272458713573));
#6217=CARTESIAN_POINT('Ctrl Pts',(-26.4120572689161,-1.22888610491339,2.73677701321046));
#6218=CARTESIAN_POINT('Ctrl Pts',(-26.4465442238038,-1.21000802381102,2.74517577574546));
#6219=CARTESIAN_POINT('Ctrl Pts',(-26.4635468416444,-1.20010753017731,2.74952213668882));
#6220=CARTESIAN_POINT('Ctrl Pts',(-26.4970804298005,-1.17938992628659,2.75847230162352));
#6221=CARTESIAN_POINT('Ctrl Pts',(-26.5136113919084,-1.16857280798542,2.76307612855274));
#6222=CARTESIAN_POINT('Ctrl Pts',(-26.5462078840406,-1.14602038731631,2.77250596727389));
#6223=CARTESIAN_POINT('Ctrl Pts',(-26.562273493867,-1.1342850254395,2.7773320282384));
#6224=CARTESIAN_POINT('Ctrl Pts',(-26.5939414283119,-1.1098870091199,2.78717177677759));
#6225=CARTESIAN_POINT('Ctrl Pts',(-26.6095473445416,-1.09722131473955,2.79218666030944));
#6226=CARTESIAN_POINT('Ctrl Pts',(-26.6402811143626,-1.07095661488449,2.8023656091679));
#6227=CARTESIAN_POINT('Ctrl Pts',(-26.6552948463125,-1.0574557506976,2.80749156457345));
#6228=CARTESIAN_POINT('Ctrl Pts',(-26.6846546110444,-1.02971343125001,2.817784903976));
#6229=CARTESIAN_POINT('Ctrl Pts',(-26.6989977054847,-1.0154744409772,2.82295134426973));
#6230=CARTESIAN_POINT('Ctrl Pts',(-26.7270250638549,-0.98626566630943,2.83328830718172));
#6231=CARTESIAN_POINT('Ctrl Pts',(-26.7407092830319,-0.971295850373591,
2.83845888576662));
#6232=CARTESIAN_POINT('Ctrl Pts',(-26.7807869864753,-0.925288343298035,
2.85392552592912));
#6233=CARTESIAN_POINT('Ctrl Pts',(-26.8062104528913,-0.893151438987829,
2.86417785822885));
#6234=CARTESIAN_POINT('Ctrl Pts',(-26.8423944800688,-0.842704105273581,
2.87926390500452));
#6235=CARTESIAN_POINT('Ctrl Pts',(-26.854135591242,-0.825504489114962,2.88424645343755));
#6236=CARTESIAN_POINT('Ctrl Pts',(-26.8712462612575,-0.799138658144533,
2.89161951102431));
#6237=CARTESIAN_POINT('Ctrl Pts',(-26.876870779104,-0.790247883055737,2.89406240563577));
#6238=CARTESIAN_POINT('Ctrl Pts',(-26.8879469072246,-0.772281655830627,
2.89890846334945));
#6239=CARTESIAN_POINT('Ctrl Pts',(-26.893409269784,-0.763187520111312,2.90131641792487));
#6240=CARTESIAN_POINT('Ctrl Pts',(-26.9094749238114,-0.735724555729972,
2.90844791977076));
#6241=CARTESIAN_POINT('Ctrl Pts',(-26.9197549867311,-0.717184843056228,
2.91307769758814));
#6242=CARTESIAN_POINT('Ctrl Pts',(-26.9394913365264,-0.679605859000123,
2.92207317082987));
#6243=CARTESIAN_POINT('Ctrl Pts',(-26.9489438557812,-0.660573303647308,
2.92643722327291));
#6244=CARTESIAN_POINT('Ctrl Pts',(-26.9760661551845,-0.602745633656236,
2.93909124911831));
#6245=CARTESIAN_POINT('Ctrl Pts',(-26.9925036507446,-0.563222175536769,
2.94694362837257));
#6246=CARTESIAN_POINT('Ctrl Pts',(-27.0220715762404,-0.482184664459269,
2.96128235245645));
#6247=CARTESIAN_POINT('Ctrl Pts',(-27.0352035249924,-0.440658030285012,
2.96777002657001));
#6248=CARTESIAN_POINT('Ctrl Pts',(-27.0523216883035,-0.376833839229866,
2.97631699067074));
#6249=CARTESIAN_POINT('Ctrl Pts',(-27.0576005303158,-0.355274412887369,
2.97897027612799));
#6250=CARTESIAN_POINT('Ctrl Pts',(-27.0672600591522,-0.311662753136127,
2.98384821443584));
#6251=CARTESIAN_POINT('Ctrl Pts',(-27.0716114828177,-0.289741794867057,
2.9860580250039));
#6252=CARTESIAN_POINT('Ctrl Pts',(-27.0793660357628,-0.245626078050731,
2.99001014183974));
#6253=CARTESIAN_POINT('Ctrl Pts',(-27.0827661298392,-0.223449095191076,
2.99175090619715));
#6254=CARTESIAN_POINT('Ctrl Pts',(-27.088612570746,-0.178789136156301,2.99475173451271));
#6255=CARTESIAN_POINT('Ctrl Pts',(-27.0910448696872,-0.1564046715903,2.99600458388059));
#6256=CARTESIAN_POINT('Ctrl Pts',(-27.096853679446,-0.0893800225646477,
2.9990010619891));
#6257=CARTESIAN_POINT('Ctrl Pts',(-27.098776248484,-0.0447217666279726,
2.99999873125252));
#6258=CARTESIAN_POINT('Ctrl Pts',(-27.0987810099015,0.0221932423036746,
3.00000122002206));
#6259=CARTESIAN_POINT('Ctrl Pts',(-27.0983026039981,0.0444881794306487,
2.99975332625577));
#6260=CARTESIAN_POINT('Ctrl Pts',(-27.0963847740834,0.0890579105479431,
2.99876106205554));
#6261=CARTESIAN_POINT('Ctrl Pts',(-27.0949453773135,0.111332705013246,2.99801669216856));
#6262=CARTESIAN_POINT('Ctrl Pts',(-27.0910975380372,0.155862012281645,2.99603172453301));
#6263=CARTESIAN_POINT('Ctrl Pts',(-27.0886879051299,0.178121225730192,2.99479051237394));
#6264=CARTESIAN_POINT('Ctrl Pts',(-27.0828889596371,0.222600296296532,2.99181384430896));
#6265=CARTESIAN_POINT('Ctrl Pts',(-27.0794840506901,0.244888396742269,2.99007048023225));
#6266=CARTESIAN_POINT('Ctrl Pts',(-27.071775952777,0.288869899263917,2.98614166251469));
#6267=CARTESIAN_POINT('Ctrl Pts',(-27.0674608269688,0.310670331278556,2.98395006519914));
#6268=CARTESIAN_POINT('Ctrl Pts',(-27.0579363802439,0.353839366034685,2.9791394357373));
#6269=CARTESIAN_POINT('Ctrl Pts',(-27.0527258255725,0.375218389994932,2.97651976178013));
#6270=CARTESIAN_POINT('Ctrl Pts',(-27.0357695640527,0.438751704381788,2.96805078583667));
#6271=CARTESIAN_POINT('Ctrl Pts',(-27.0226990393997,0.48031037316965,2.96158999423889));
#6272=CARTESIAN_POINT('Ctrl Pts',(-27.0004754778274,0.541446390227552,2.95080792183841));
#6273=CARTESIAN_POINT('Ctrl Pts',(-26.9926233391618,0.561639756422948,2.94702858491465));
#6274=CARTESIAN_POINT('Ctrl Pts',(-26.9801906409175,0.5916140025928,2.94110512698185));
#6275=CARTESIAN_POINT('Ctrl Pts',(-26.9759329233523,0.601561926835117,2.9390861971729));
#6276=CARTESIAN_POINT('Ctrl Pts',(-26.9671986892834,0.621350277064186,2.93496653895837));
#6277=CARTESIAN_POINT('Ctrl Pts',(-26.9627160190823,0.631203054805755,2.93286297248301));
#6278=CARTESIAN_POINT('Ctrl Pts',(-26.949000010224,0.660466243653672,2.92646286445819));
#6279=CARTESIAN_POINT('Ctrl Pts',(-26.9394863006083,0.679616625492281,2.92207081256718));
#6280=CARTESIAN_POINT('Ctrl Pts',(-26.9197260539462,0.717238752620466,2.91306457362862));
#6281=CARTESIAN_POINT('Ctrl Pts',(-26.9094809907086,0.7357078120015,2.90845102679016));
#6282=CARTESIAN_POINT('Ctrl Pts',(-26.8776648850953,0.790113953263617,2.8943267049494));
#6283=CARTESIAN_POINT('Ctrl Pts',(-26.8550156533739,0.825052204528997,2.88453180649776));
#6284=CARTESIAN_POINT('Ctrl Pts',(-26.8188825262082,0.875510966128809,2.86945837323707));
#6285=CARTESIAN_POINT('Ctrl Pts',(-26.8064775830923,0.892005171014219,2.86437028648305));
#6286=CARTESIAN_POINT('Ctrl Pts',(-26.7809368156929,0.92434327478541,2.85409879125165));
#6287=CARTESIAN_POINT('Ctrl Pts',(-26.767806005017,0.940181255880788,2.8489172911309));
#6288=CARTESIAN_POINT('Ctrl Pts',(-26.7475346890206,0.963464821076118,2.84109226874023));
#6289=CARTESIAN_POINT('Ctrl Pts',(-26.7406844898386,0.971142790692541,2.83847640424403));
#6290=CARTESIAN_POINT('Ctrl Pts',(-26.7268665710498,0.986257223502056,2.83326015443131));
#6291=CARTESIAN_POINT('Ctrl Pts',(-26.7198861854429,0.993708406579356,2.83065485672359));
#6292=CARTESIAN_POINT('Ctrl Pts',(-26.6987543184742,1.01572209996892,2.82286262012559));
#6293=CARTESIAN_POINT('Ctrl Pts',(-26.6843926989096,1.02996746343674,2.81769174714818));
#6294=CARTESIAN_POINT('Ctrl Pts',(-26.6405194665222,1.07140391340386,2.80231410558904));
#6295=CARTESIAN_POINT('Ctrl Pts',(-26.6101987968579,1.09732460419766,2.79223276559478));
#6296=CARTESIAN_POINT('Ctrl Pts',(-26.5630918828768,1.13367250400702,2.77758169296716));
#6297=CARTESIAN_POINT('Ctrl Pts',(-26.5471174957754,1.14536614557726,2.7727762680603));
#6298=CARTESIAN_POINT('Ctrl Pts',(-26.514612671107,1.16790354588699,2.76335903848249));
#6299=CARTESIAN_POINT('Ctrl Pts',(-26.4980822787532,1.17874735889937,2.7587471803173));
#6300=CARTESIAN_POINT('Ctrl Pts',(-26.46444880388,1.19957259205024,2.74975580028195));
#6301=CARTESIAN_POINT('Ctrl Pts',(-26.4473524929256,1.20955009125368,2.74537799392286));
#6302=CARTESIAN_POINT('Ctrl Pts',(-26.4212416835811,1.22386590602098,2.73901119026752));
#6303=CARTESIAN_POINT('Ctrl Pts',(-26.4124619953677,1.22852739949808,2.73692306012723));
#6304=CARTESIAN_POINT('Ctrl Pts',(-26.3948577516024,1.23757286419293,2.73284480288515));
#6305=CARTESIAN_POINT('Ctrl Pts',(-26.3860147393496,1.2419677956983,2.73084989444486));
#6306=CARTESIAN_POINT('Ctrl Pts',(-26.3416451282571,1.26327195668703,2.72112034953697));
#6307=CARTESIAN_POINT('Ctrl Pts',(-26.3055754632133,1.27824521948246,2.71409222828943));
#6308=CARTESIAN_POINT('Ctrl Pts',(-26.2323060083433,1.30407984829821,2.70177412725945));
#6309=CARTESIAN_POINT('Ctrl Pts',(-26.1951016228418,1.31494638090081,2.69648191406169));
#6310=CARTESIAN_POINT('Ctrl Pts',(-26.1384100565222,1.3281154276414,2.69000670173171));
#6311=CARTESIAN_POINT('Ctrl Pts',(-26.1193651709025,1.33198245867611,2.68809214937698));
#6312=CARTESIAN_POINT('Ctrl Pts',(-26.0809718351375,1.33864905018687,2.68477846139787));
#6313=CARTESIAN_POINT('Ctrl Pts',(-26.0616267046488,1.34144791557871,2.68337970984735));
#6314=CARTESIAN_POINT('Ctrl Pts',(-26.0323637266099,1.34482464575181,2.68168810040418));
#6315=CARTESIAN_POINT('Ctrl Pts',(-26.0225572452852,1.34581322849437,2.68119198692629));
#6316=CARTESIAN_POINT('Ctrl Pts',(-26.0029866629929,1.34750144912674,2.68034392500147));
#6317=CARTESIAN_POINT('Ctrl Pts',(-25.993207230682,1.34820337332278,2.67999083517032));
#6318=CARTESIAN_POINT('Ctrl Pts',(-25.9639248638171,1.34988238530037,2.67914574940457));
#6319=CARTESIAN_POINT('Ctrl Pts',(-25.944430250381,1.35043878696276,2.67886501715933));
#6320=CARTESIAN_POINT('Ctrl Pts',(-25.8861245564454,1.35043705000303,2.67886596390228));
#6321=CARTESIAN_POINT('Ctrl Pts',(-25.8474104061639,1.34822092631381,2.67998650091244));
#6322=CARTESIAN_POINT('Ctrl Pts',(-25.7896109432291,1.34160967645963,2.68329876772693));
#6323=CARTESIAN_POINT('Ctrl Pts',(-25.7703875060739,1.33885738792583,2.68467452923362));
#6324=CARTESIAN_POINT('Ctrl Pts',(-25.7320267909422,1.33224993750147,2.68795954661436));
#6325=CARTESIAN_POINT('Ctrl Pts',(-25.7128830927771,1.32839290578458,2.68986973704837));
#6326=CARTESIAN_POINT('Ctrl Pts',(-25.684251825295,1.32177548884068,2.69312428914529));
#6327=CARTESIAN_POINT('Ctrl Pts',(-25.6747142093514,1.31942848978327,2.69427521202406));
#6328=CARTESIAN_POINT('Ctrl Pts',(-25.6556603366635,1.31445289803521,2.6967061495634));
#6329=CARTESIAN_POINT('Ctrl Pts',(-25.6461500334678,1.31182518416256,2.69798570492286));
#6330=CARTESIAN_POINT('Ctrl Pts',(-25.6178200674555,1.30356617188208,2.70199101363685));
#6331=CARTESIAN_POINT('Ctrl Pts',(-25.5991463885073,1.2975477717278,2.70488904077814));
#6332=CARTESIAN_POINT('Ctrl Pts',(-25.5622143033361,1.28450992377734,2.711104791713));
#6333=CARTESIAN_POINT('Ctrl Pts',(-25.5439552645306,1.27749068571576,2.7144224184567));
#6334=CARTESIAN_POINT('Ctrl Pts',(-25.5078400226815,1.26246775944474,2.72144201858098));
#6335=CARTESIAN_POINT('Ctrl Pts',(-25.4899838433394,1.25446401700334,2.72514402265193));
#6336=CARTESIAN_POINT('Ctrl Pts',(-25.4370074508209,1.22898778436132,2.736775538613));
#6337=CARTESIAN_POINT('Ctrl Pts',(-25.402476169391,1.21005033530758,2.74523167785092));
#6338=CARTESIAN_POINT('Ctrl Pts',(-25.3602840547609,1.18392811236616,2.75651044711871));
#6339=CARTESIAN_POINT('Ctrl Pts',(-25.3518921545878,1.17857779567387,2.75880270804698));
#6340=CARTESIAN_POINT('Ctrl Pts',(-25.33521027166,1.16763346103172,2.76345258994632));
#6341=CARTESIAN_POINT('Ctrl Pts',(-25.3269101970962,1.16203150593468,2.76581339519711));
#6342=CARTESIAN_POINT('Ctrl Pts',(-25.3022697723606,1.14492960216065,2.77295715687365));
#6343=CARTESIAN_POINT('Ctrl Pts',(-25.2861659342133,1.13312196993095,2.77780680847141));
#6344=CARTESIAN_POINT('Ctrl Pts',(-25.2545677370148,1.10869517847092,2.78764614588441));
#6345=CARTESIAN_POINT('Ctrl Pts',(-25.2390760976615,1.09607817216592,2.79263498420858));
#6346=CARTESIAN_POINT('Ctrl Pts',(-25.2086929585038,1.0700438882078,2.80271360615569));
#6347=CARTESIAN_POINT('Ctrl Pts',(-25.1938014786094,1.05662659440153,2.80780342156985));
#6348=CARTESIAN_POINT('Ctrl Pts',(-25.1646092945331,1.02899172455791,2.81804822663801));
#6349=CARTESIAN_POINT('Ctrl Pts',(-25.1503085987059,1.01477414783796,2.82320324630945));
#6350=CARTESIAN_POINT('Ctrl Pts',(-25.122293720064,0.985531953026374,2.83354369456913));
#6351=CARTESIAN_POINT('Ctrl Pts',(-25.1085795345898,0.970507349552267,2.83872915299999));
#6352=CARTESIAN_POINT('Ctrl Pts',(-25.0817384653232,0.939637469740702,2.84909618968299));
#6353=CARTESIAN_POINT('Ctrl Pts',(-25.0686121956922,0.923792524689849,2.85427759753642));
#6354=CARTESIAN_POINT('Ctrl Pts',(-25.0493658734545,0.899393021425867,2.86202163910769));
#6355=CARTESIAN_POINT('Ctrl Pts',(-25.043017487774,0.891144418134318,2.86460120904708));
#6356=CARTESIAN_POINT('Ctrl Pts',(-25.0305207080604,0.874501431709212,2.86972568743743));
#6357=CARTESIAN_POINT('Ctrl Pts',(-25.0243713909441,0.866107457626742,2.87227076450331));
#6358=CARTESIAN_POINT('Ctrl Pts',(-24.9941176023294,0.823767677123202,2.88490127988302));
#6359=CARTESIAN_POINT('Ctrl Pts',(-24.97147225811,0.788728779396098,2.89470358965755));
#6360=CARTESIAN_POINT('Ctrl Pts',(-24.9292312229828,0.716311799075428,2.9134684860099));
#6361=CARTESIAN_POINT('Ctrl Pts',(-24.9096337112948,0.67893447464684,2.92243229488295));
#6362=CARTESIAN_POINT('Ctrl Pts',(-24.8825415051001,0.621060303181761,2.93507687968496));
#6363=CARTESIAN_POINT('Ctrl Pts',(-24.8738954614447,0.601467085362858,2.93915828390893));
#6364=CARTESIAN_POINT('Ctrl Pts',(-24.8573860335644,0.561660534816686,2.94702417229759));
#6365=CARTESIAN_POINT('Ctrl Pts',(-24.8495222347111,0.541445118061444,2.95080889756673));
#6366=CARTESIAN_POINT('Ctrl Pts',(-24.8383296294352,0.510647204231347,2.95623934885628));
#6367=CARTESIAN_POINT('Ctrl Pts',(-24.8346943538624,0.500285572119667,2.95801084324021));
#6368=CARTESIAN_POINT('Ctrl Pts',(-24.8276507980447,0.479467813925561,2.96145644444383));
#6369=CARTESIAN_POINT('Ctrl Pts',(-24.8242486897808,0.469031540585877,2.96312749437884));
#6370=CARTESIAN_POINT('Ctrl Pts',(-24.8143975220266,0.437635545407865,2.967983313185));
#6371=CARTESIAN_POINT('Ctrl Pts',(-24.8082918810615,0.41655941359351,2.97101630939715));
#6372=CARTESIAN_POINT('Ctrl Pts',(-24.79700967936,0.374165575587154,2.97665244169902));
#6373=CARTESIAN_POINT('Ctrl Pts',(-24.7918302021315,0.352839925216633,2.97925701409689));
#6374=CARTESIAN_POINT('Ctrl Pts',(-24.782389529693,0.309931149531077,2.98402597733368));
#6375=CARTESIAN_POINT('Ctrl Pts',(-24.7781283401501,0.288348024079468,2.98619038155605));
#6376=CARTESIAN_POINT('Ctrl Pts',(-24.7705262413241,0.244922587990788,2.99006529803462));
#6377=CARTESIAN_POINT('Ctrl Pts',(-24.767185323199,0.223080280695768,2.9917758240911));
#6378=CARTESIAN_POINT('Ctrl Pts',(-24.7614327168412,0.179133051352736,2.99472848957151));
#6379=CARTESIAN_POINT('Ctrl Pts',(-24.7590210045444,0.157028136357561,2.9959706439119));
#6380=CARTESIAN_POINT('Ctrl Pts',(-24.7551430015195,0.112550450866727,2.99797103284412));
#6381=CARTESIAN_POINT('Ctrl Pts',(-24.7536770371529,0.0901765544388111,
2.99872909299962));
#6382=CARTESIAN_POINT('Ctrl Pts',(-24.7522040612047,0.056412819484831,2.9994911778993));
#6383=CARTESIAN_POINT('Ctrl Pts',(-24.7518343852008,0.0451068922413156,
2.999682558101));
#6384=CARTESIAN_POINT('Ctrl Pts',(-24.7513427166217,0.0225174680468748,
2.99993712712975));
#6385=CARTESIAN_POINT('Ctrl Pts',(-24.7512203639079,0.0112452244724433,
3.00000050164314));
#6386=CARTESIAN_POINT('Ctrl Pts',(-24.7512205732181,-1.76183185122132E-16,
3.00000039251396));
#6387=CARTESIAN_POINT('Ctrl Pts',(-24.925,1.55854062294791E-16,2.60755260924175));
#6388=CARTESIAN_POINT('Ctrl Pts',(-24.9250003566431,-0.0166541858892895,
2.60755241953505));
#6389=CARTESIAN_POINT('Ctrl Pts',(-24.9254160783661,-0.0332581559508135,
2.60733265858179));
#6390=CARTESIAN_POINT('Ctrl Pts',(-24.9270649354643,-0.0663304974791156,
2.60646231020683));
#6391=CARTESIAN_POINT('Ctrl Pts',(-24.9282977615931,-0.0828051219601001,
2.60581189691127));
#6392=CARTESIAN_POINT('Ctrl Pts',(-24.9332076090917,-0.132046707858214,
2.60322787601199));
#6393=CARTESIAN_POINT('Ctrl Pts',(-24.9380956117425,-0.164639289236404,
2.6006604794867));
#6394=CARTESIAN_POINT('Ctrl Pts',(-24.9478395671871,-0.213143553563254,
2.59559297392188));
#6395=CARTESIAN_POINT('Ctrl Pts',(-24.9514952030343,-0.229263645988799,
2.59369843168223));
#6396=CARTESIAN_POINT('Ctrl Pts',(-24.9575851418319,-0.253332291674963,
2.59055979222183));
#6397=CARTESIAN_POINT('Ctrl Pts',(-24.9597188141185,-0.261344691370318,
2.58946279377859));
#6398=CARTESIAN_POINT('Ctrl Pts',(-24.9641906612921,-0.277334518444499,
2.58717039663941));
#6399=CARTESIAN_POINT('Ctrl Pts',(-24.966530765891,-0.285316779266169,2.58597403111897));
#6400=CARTESIAN_POINT('Ctrl Pts',(-24.973820513222,-0.309081961524915,2.58225915775743));
#6401=CARTESIAN_POINT('Ctrl Pts',(-24.9790484377681,-0.324723793798948,
2.57961022574372));
#6402=CARTESIAN_POINT('Ctrl Pts',(-24.9902256908821,-0.355621851323135,
2.57399040352469));
#6403=CARTESIAN_POINT('Ctrl Pts',(-24.9961745187184,-0.37087717201515,2.57101975041036));
#6404=CARTESIAN_POINT('Ctrl Pts',(-25.0150836576248,-0.416076046241271,
2.5616604629974));
#6405=CARTESIAN_POINT('Ctrl Pts',(-25.0291043543913,-0.445453982261499,
2.5548242940218));
#6406=CARTESIAN_POINT('Ctrl Pts',(-25.0522383184702,-0.488417442273932,
2.54380826092923));
#6407=CARTESIAN_POINT('Ctrl Pts',(-25.0603014453932,-0.502555351656382,
2.54000886254707));
#6408=CARTESIAN_POINT('Ctrl Pts',(-25.0771344181921,-0.530461627229323,
2.53217843551044));
#6409=CARTESIAN_POINT('Ctrl Pts',(-25.0859109306211,-0.544239963564881,
2.52814434334757));
#6410=CARTESIAN_POINT('Ctrl Pts',(-25.1041597996001,-0.571392063284267,
2.51987677295435));
#6411=CARTESIAN_POINT('Ctrl Pts',(-25.1135652356457,-0.584667955785163,
2.51567359591458));
#6412=CARTESIAN_POINT('Ctrl Pts',(-25.1329503931644,-0.610672109363501,
2.50714732573442));
#6413=CARTESIAN_POINT('Ctrl Pts',(-25.1429262744659,-0.623394578020972,
2.50282595067223));
#6414=CARTESIAN_POINT('Ctrl Pts',(-25.1736949347874,-0.660743188336079,
2.48973044146157));
#6415=CARTESIAN_POINT('Ctrl Pts',(-25.1953265696652,-0.684552408790031,
2.48082441641631));
#6416=CARTESIAN_POINT('Ctrl Pts',(-25.2294621790932,-0.718669526189459,
2.46737442476458));
#6417=CARTESIAN_POINT('Ctrl Pts',(-25.2411226141971,-0.729775262858415,
2.46287588038062));
#6418=CARTESIAN_POINT('Ctrl Pts',(-25.2650163395357,-0.751453108570394,
2.45387816269178));
#6419=CARTESIAN_POINT('Ctrl Pts',(-25.2772554632753,-0.762029504500183,
2.44937698167527));
#6420=CARTESIAN_POINT('Ctrl Pts',(-25.3022971286316,-0.782626892006877,
2.44041267983556));
#6421=CARTESIAN_POINT('Ctrl Pts',(-25.315157197433,-0.792689421921387,2.43593042229927));
#6422=CARTESIAN_POINT('Ctrl Pts',(-25.341232755504,-0.812083164942917,2.42711283865451));
#6423=CARTESIAN_POINT('Ctrl Pts',(-25.3544672859955,-0.821434074532997,
2.42276972387511));
#6424=CARTESIAN_POINT('Ctrl Pts',(-25.3813264071519,-0.839452527788181,
2.41424554238549));
#6425=CARTESIAN_POINT('Ctrl Pts',(-25.3949513697869,-0.848120793930842,
2.41006421940509));
#6426=CARTESIAN_POINT('Ctrl Pts',(-25.4225940554056,-0.864782458141236,
2.40189271204072));
#6427=CARTESIAN_POINT('Ctrl Pts',(-25.4366117834694,-0.872775835903153,
2.39790249830954));
#6428=CARTESIAN_POINT('Ctrl Pts',(-25.479261734589,-0.895745723912417,2.386263986526));
#6429=CARTESIAN_POINT('Ctrl Pts',(-25.5084958123966,-0.909716954879009,
2.3789457429218));
#6430=CARTESIAN_POINT('Ctrl Pts',(-25.5535776615725,-0.928607298291761,
2.36882679203486));
#6431=CARTESIAN_POINT('Ctrl Pts',(-25.5688253899689,-0.934563660377399,
2.36559439343673));
#6432=CARTESIAN_POINT('Ctrl Pts',(-25.5920023693806,-0.942963605388763,
2.36098892152975));
#6433=CARTESIAN_POINT('Ctrl Pts',(-25.5997879839068,-0.94567716643989,2.35949277008249));
#6434=CARTESIAN_POINT('Ctrl Pts',(-25.6154612044865,-0.950922793268216,
2.35658631440842));
#6435=CARTESIAN_POINT('Ctrl Pts',(-25.6233613960042,-0.953458374961467,
2.35517402568802));
#6436=CARTESIAN_POINT('Ctrl Pts',(-25.6470876486476,-0.960748669979318,
2.35109499689056));
#6437=CARTESIAN_POINT('Ctrl Pts',(-25.6629694924038,-0.965199959788432,
2.34857921219019));
#6438=CARTESIAN_POINT('Ctrl Pts',(-25.6948784413748,-0.973301096108641,
2.34396841563555));
#6439=CARTESIAN_POINT('Ctrl Pts',(-25.710902645268,-0.976950283068506,2.34187376666204));
#6440=CARTESIAN_POINT('Ctrl Pts',(-25.7591844222772,-0.986703415822536,
2.33624500537071));
#6441=CARTESIAN_POINT('Ctrl Pts',(-25.791650783833,-0.991615665333941,2.33336629059962));
#6442=CARTESIAN_POINT('Ctrl Pts',(-25.8407756179032,-0.996582697577232,
2.3304458498952));
#6443=CARTESIAN_POINT('Ctrl Pts',(-25.8572215351598,-0.997837487879419,
2.329705241771));
#6444=CARTESIAN_POINT('Ctrl Pts',(-25.8902578614934,-0.999533165226665,
2.32870354106611));
#6445=CARTESIAN_POINT('Ctrl Pts',(-25.9068578724972,-0.999973524878361,
2.32844279123645));
#6446=CARTESIAN_POINT('Ctrl Pts',(-25.940167362761,-1.0000242628141,2.32841276730314));
#6447=CARTESIAN_POINT('Ctrl Pts',(-25.9569704588412,-0.999628762374181,
2.32864698234144));
#6448=CARTESIAN_POINT('Ctrl Pts',(-25.9903233075244,-0.998003316619995,
2.32960735397222));
#6449=CARTESIAN_POINT('Ctrl Pts',(-26.0069064582144,-0.99677776727011,2.33033089082929));
#6450=CARTESIAN_POINT('Ctrl Pts',(-26.0398870987565,-0.993516757651968,
2.33224874868744));
#6451=CARTESIAN_POINT('Ctrl Pts',(-26.0562852280577,-0.991481744891029,
2.33344279183591));
#6452=CARTESIAN_POINT('Ctrl Pts',(-26.0889006503167,-0.986614637292695,
2.33628332558741));
#6453=CARTESIAN_POINT('Ctrl Pts',(-26.1051179364934,-0.983782507538745,
2.33792982096873));
#6454=CARTESIAN_POINT('Ctrl Pts',(-26.1535021710044,-0.974099057442964,
2.34352095101131));
#6455=CARTESIAN_POINT('Ctrl Pts',(-26.1854056292135,-0.966060458399386,
2.3481189625644));
#6456=CARTESIAN_POINT('Ctrl Pts',(-26.2248342916283,-0.954027413144459,
2.35485651240159));
#6457=CARTESIAN_POINT('Ctrl Pts',(-26.2327013987641,-0.951518784920255,
2.35625480890824));
#6458=CARTESIAN_POINT('Ctrl Pts',(-26.2483827345867,-0.946304393522068,
2.35914625498642));
#6459=CARTESIAN_POINT('Ctrl Pts',(-26.2562117486977,-0.94359270504545,2.36064260344912));
#6460=CARTESIAN_POINT('Ctrl Pts',(-26.2795250530157,-0.935192248164096,
2.3652521259866));
#6461=CARTESIAN_POINT('Ctrl Pts',(-26.2948382163531,-0.929240340102424,
2.36848474521895));
#6462=CARTESIAN_POINT('Ctrl Pts',(-26.325052120344,-0.916638547977859,2.37524073173657));
#6463=CARTESIAN_POINT('Ctrl Pts',(-26.3399478665267,-0.90999062203962,2.37876303600403));
#6464=CARTESIAN_POINT('Ctrl Pts',(-26.3693289871196,-0.896011395896082,
2.38606310676974));
#6465=CARTESIAN_POINT('Ctrl Pts',(-26.3838143473607,-0.888680076643438,
2.38984089454833));
#6466=CARTESIAN_POINT('Ctrl Pts',(-26.4123832482896,-0.873338683184522,
2.3976202355067));
#6467=CARTESIAN_POINT('Ctrl Pts',(-26.4264667819849,-0.865328603021505,
2.40162180862374));
#6468=CARTESIAN_POINT('Ctrl Pts',(-26.4542373250601,-0.848628527049356,
2.40981807440537));
#6469=CARTESIAN_POINT('Ctrl Pts',(-26.4679244024272,-0.839938487173806,
2.41401280980997));
#6470=CARTESIAN_POINT('Ctrl Pts',(-26.4949038618746,-0.821871746929689,
2.42256536268358));
#6471=CARTESIAN_POINT('Ctrl Pts',(-26.5081993038235,-0.812492795486007,
2.42692421965941));
#6472=CARTESIAN_POINT('Ctrl Pts',(-26.5343829028199,-0.793043775382972,
2.43577160005359));
#6473=CARTESIAN_POINT('Ctrl Pts',(-26.5471738340693,-0.7830463803841,2.44022699893486));
#6474=CARTESIAN_POINT('Ctrl Pts',(-26.5721868510483,-0.762503182417991,
2.4491738057699));
#6475=CARTESIAN_POINT('Ctrl Pts',(-26.5844064334615,-0.751959204775381,
2.45366439347184));
#6476=CARTESIAN_POINT('Ctrl Pts',(-26.6082843084103,-0.730330096168273,
2.46264911716722));
#6477=CARTESIAN_POINT('Ctrl Pts',(-26.6199425628188,-0.719244941847823,
2.46714330180598));
#6478=CARTESIAN_POINT('Ctrl Pts',(-26.6540867150583,-0.685176365586002,
2.48058665935111));
#6479=CARTESIAN_POINT('Ctrl Pts',(-26.6757462073237,-0.661378975879618,
2.48949782346477));
#6480=CARTESIAN_POINT('Ctrl Pts',(-26.706573146655,-0.624022706324938,2.50261037529357));
#6481=CARTESIAN_POINT('Ctrl Pts',(-26.7165759724886,-0.611286384102542,
2.50694112711597));
#6482=CARTESIAN_POINT('Ctrl Pts',(-26.7311533876529,-0.591762476370502,
2.51334967146033));
#6483=CARTESIAN_POINT('Ctrl Pts',(-26.7359451890069,-0.585178854079478,
2.51547299658858));
#6484=CARTESIAN_POINT('Ctrl Pts',(-26.7453814833122,-0.571874856074331,
2.51968511284943));
#6485=CARTESIAN_POINT('Ctrl Pts',(-26.7500351366602,-0.565140645160058,
2.52177806865428));
#6486=CARTESIAN_POINT('Ctrl Pts',(-26.7637222516845,-0.544804309725444,
2.52797665659196));
#6487=CARTESIAN_POINT('Ctrl Pts',(-26.7724803391795,-0.531075645530332,
2.53200078580808));
#6488=CARTESIAN_POINT('Ctrl Pts',(-26.7892946991393,-0.503248393728809,
2.53981950802605));
#6489=CARTESIAN_POINT('Ctrl Pts',(-26.7973477617837,-0.489154779345306,
2.54361267297453));
#6490=CARTESIAN_POINT('Ctrl Pts',(-26.8204545728125,-0.446333368005571,
2.55461135090607));
#6491=CARTESIAN_POINT('Ctrl Pts',(-26.834458477791,-0.417066232433276,2.56143651401679));
#6492=CARTESIAN_POINT('Ctrl Pts',(-26.8596488370896,-0.357057925052845,
2.57389950485307));
#6493=CARTESIAN_POINT('Ctrl Pts',(-26.8708365853539,-0.326307436876508,
2.57953848796632));
#6494=CARTESIAN_POINT('Ctrl Pts',(-26.8854203844307,-0.279045599412756,
2.58696737317913));
#6495=CARTESIAN_POINT('Ctrl Pts',(-26.8899176876621,-0.263080836121057,
2.58927356668171));
#6496=CARTESIAN_POINT('Ctrl Pts',(-26.8981471118759,-0.230786385702436,
2.59351339304777));
#6497=CARTESIAN_POINT('Ctrl Pts',(-26.901854302142,-0.214553907874612,2.59543412523402));
#6498=CARTESIAN_POINT('Ctrl Pts',(-26.9084607843892,-0.181886203010055,
2.59886924230702));
#6499=CARTESIAN_POINT('Ctrl Pts',(-26.9113574905324,-0.165464138876776,
2.6003822869898));
#6500=CARTESIAN_POINT('Ctrl Pts',(-26.9163383589761,-0.132393422445163,
2.60299055921658));
#6501=CARTESIAN_POINT('Ctrl Pts',(-26.9184105531932,-0.1158177180384,2.60407951595309));
#6502=CARTESIAN_POINT('Ctrl Pts',(-26.9233593618272,-0.0661859402484176,
2.60668400705037));
#6503=CARTESIAN_POINT('Ctrl Pts',(-26.9249972922528,-0.0331164849794928,
2.60755116529974));
#6504=CARTESIAN_POINT('Ctrl Pts',(-26.9250013487368,0.016434104258675,2.60755332849863));
#6505=CARTESIAN_POINT('Ctrl Pts',(-26.924593771391,0.0329435135702283,2.60733786318112));
#6506=CARTESIAN_POINT('Ctrl Pts',(-26.9229598784543,0.0659474161951004,
2.60647540292584));
#6507=CARTESIAN_POINT('Ctrl Pts',(-26.9217335860717,0.0824419098590674,
2.60582840846348));
#6508=CARTESIAN_POINT('Ctrl Pts',(-26.9184554239328,0.115415878608658,2.60410310617677));
#6509=CARTESIAN_POINT('Ctrl Pts',(-26.9164025400161,0.131898834522029,2.60302426431673));
#6510=CARTESIAN_POINT('Ctrl Pts',(-26.9114621352338,0.164835602978561,2.60043699179505));
#6511=CARTESIAN_POINT('Ctrl Pts',(-26.9085613270678,0.181339949722123,2.59892168747799));
#6512=CARTESIAN_POINT('Ctrl Pts',(-26.9019944221297,0.213908268855232,2.59550682162746));
#6513=CARTESIAN_POINT('Ctrl Pts',(-26.8983181557807,0.230051496944321,2.59360192011072));
#6514=CARTESIAN_POINT('Ctrl Pts',(-26.8902038146127,0.262018183387905,2.58942059752269));
#6515=CARTESIAN_POINT('Ctrl Pts',(-26.8857646886985,0.27784935865575,2.58714361859994));
#6516=CARTESIAN_POINT('Ctrl Pts',(-26.8713188216695,0.324895801813618,2.57978251945633));
#6517=CARTESIAN_POINT('Ctrl Pts',(-26.8601834035885,0.355670011650616,2.5741669021953));
#6518=CARTESIAN_POINT('Ctrl Pts',(-26.8412500664846,0.400941255234932,2.56479529641426));
#6519=CARTESIAN_POINT('Ctrl Pts',(-26.8345604461981,0.415894450482944,2.56151035689196));
#6520=CARTESIAN_POINT('Ctrl Pts',(-26.8239684235737,0.438090391025238,2.55636178150267));
#6521=CARTESIAN_POINT('Ctrl Pts',(-26.8203410661095,0.44545683266115,2.55460695983525));
#6522=CARTESIAN_POINT('Ctrl Pts',(-26.8128999456829,0.460110113434811,2.55102621846157));
#6523=CARTESIAN_POINT('Ctrl Pts',(-26.8090809400854,0.467406099051343,2.54919783195029));
#6524=CARTESIAN_POINT('Ctrl Pts',(-26.7973956024953,0.489075501379372,2.54363495988492));
#6525=CARTESIAN_POINT('Ctrl Pts',(-26.7892904087949,0.503256366320305,2.53981745826164));
#6526=CARTESIAN_POINT('Ctrl Pts',(-26.7724556899274,0.531115565582863,2.53198937867128));
#6527=CARTESIAN_POINT('Ctrl Pts',(-26.7637274203706,0.544791910987857,2.5279793571639));
#6528=CARTESIAN_POINT('Ctrl Pts',(-26.7366217266702,0.58507967901888,2.51570272134659));
#6529=CARTESIAN_POINT('Ctrl Pts',(-26.7173257403855,0.61095146719629,2.50718915145592));
#6530=CARTESIAN_POINT('Ctrl Pts',(-26.6865421652591,0.648316199104956,2.49408756309351));
#6531=CARTESIAN_POINT('Ctrl Pts',(-26.6759737885839,0.660530164014685,2.48966507904171));
#6532=CARTESIAN_POINT('Ctrl Pts',(-26.6542143618837,0.684476541997761,2.48073725881267));
#6533=CARTESIAN_POINT('Ctrl Pts',(-26.6430275831957,0.696204572944761,2.47623358134869));
#6534=CARTESIAN_POINT('Ctrl Pts',(-26.625757459411,0.71344606171305,2.46943219638785));
#6535=CARTESIAN_POINT('Ctrl Pts',(-26.619921440287,0.719131601096507,2.46715852858783));
#6536=CARTESIAN_POINT('Ctrl Pts',(-26.6081492806517,0.730323844266242,2.4626246472445));
#6537=CARTESIAN_POINT('Ctrl Pts',(-26.6022023493564,0.735841448132364,2.46036016392892));
#6538=CARTESIAN_POINT('Ctrl Pts',(-26.5841990801845,0.752142596351644,2.4535872758574));
#6539=CARTESIAN_POINT('Ctrl Pts',(-26.5719637153137,0.762691293347724,2.44909283533733));
#6540=CARTESIAN_POINT('Ctrl Pts',(-26.5345859666616,0.79337500010439,2.43572683396234));
#6541=CARTESIAN_POINT('Ctrl Pts',(-26.5087543078564,0.812569281368953,2.42696429363966));
#6542=CARTESIAN_POINT('Ctrl Pts',(-26.4686216279805,0.839484914822931,2.41422981442002));
#6543=CARTESIAN_POINT('Ctrl Pts',(-26.4550122677061,0.848144060795981,2.41005301554826));
#6544=CARTESIAN_POINT('Ctrl Pts',(-26.4273198206187,0.864833014186361,2.4018677094334));
#6545=CARTESIAN_POINT('Ctrl Pts',(-26.4132367723247,0.872862861793055,2.39785915569383));
#6546=CARTESIAN_POINT('Ctrl Pts',(-26.3845827730249,0.888283954759512,2.39004399122574));
#6547=CARTESIAN_POINT('Ctrl Pts',(-26.3700175910458,0.895672296665482,2.38623887159213));
#6548=CARTESIAN_POINT('Ctrl Pts',(-26.3477725177819,0.906273162875091,2.38070494715483));
#6549=CARTESIAN_POINT('Ctrl Pts',(-26.3402926727503,0.909725000544916,2.37888997766035));
#6550=CARTESIAN_POINT('Ctrl Pts',(-26.3252947580114,0.91642317054735,2.37534522135332));
#6551=CARTESIAN_POINT('Ctrl Pts',(-26.3177609641362,0.919677618978277,2.37361127867655));
#6552=CARTESIAN_POINT('Ctrl Pts',(-26.279960326246,0.935453358182173,2.36515451304933));
#6553=CARTESIAN_POINT('Ctrl Pts',(-26.2492308175849,0.946541064909445,2.35904578187965));
#6554=CARTESIAN_POINT('Ctrl Pts',(-26.1868089918217,0.965671617244593,2.3483390844543));
#6555=CARTESIAN_POINT('Ctrl Pts',(-26.1551127594127,0.973718288717797,2.3437391769445));
#6556=CARTESIAN_POINT('Ctrl Pts',(-26.1068144462703,0.983469972772359,2.33811102541253));
#6557=CARTESIAN_POINT('Ctrl Pts',(-26.090589178399,0.986333510705604,2.3364469269674));
#6558=CARTESIAN_POINT('Ctrl Pts',(-26.0578800212193,0.991270124222091,2.33356672209885));
#6559=CARTESIAN_POINT('Ctrl Pts',(-26.0413989600866,0.993342685095568,2.33235094950619));
#6560=CARTESIAN_POINT('Ctrl Pts',(-26.016468400417,0.995843155056375,2.33088062949276));
#6561=CARTESIAN_POINT('Ctrl Pts',(-26.0081137802036,0.996575200948386,2.33044941555122));
#6562=CARTESIAN_POINT('Ctrl Pts',(-25.9914406456729,0.997825328960478,2.32971229361947));
#6563=CARTESIAN_POINT('Ctrl Pts',(-25.9831090698346,0.998345104091185,2.32940539355606));
#6564=CARTESIAN_POINT('Ctrl Pts',(-25.9581619918789,0.999588413090816,2.32867085845434));
#6565=CARTESIAN_POINT('Ctrl Pts',(-25.9415535789236,1.00000042873077,2.3284268504534));
#6566=CARTESIAN_POINT('Ctrl Pts',(-25.8918801116583,0.999999142511444,2.32842767334732));
#6567=CARTESIAN_POINT('Ctrl Pts',(-25.8588976369251,0.998358102087351,2.32940162628822));
#6568=CARTESIAN_POINT('Ctrl Pts',(-25.809655452566,0.993462469088689,2.33228059590287));
#6569=CARTESIAN_POINT('Ctrl Pts',(-25.7932780679245,0.991424398396008,2.33347638591532));
#6570=CARTESIAN_POINT('Ctrl Pts',(-25.7605967018549,0.986531578876194,2.33633167075591));
#6571=CARTESIAN_POINT('Ctrl Pts',(-25.744287250752,0.983675445441529,2.3379919778889));
#6572=CARTESIAN_POINT('Ctrl Pts',(-25.7198948761487,0.978775245710681,2.34082078278938));
#6573=CARTESIAN_POINT('Ctrl Pts',(-25.7117693154796,0.97703729202741,2.34182114664376));
#6574=CARTESIAN_POINT('Ctrl Pts',(-25.6955363910876,0.973352864470024,2.34393407887515));
#6575=CARTESIAN_POINT('Ctrl Pts',(-25.6874340994824,0.971407041360756,2.34504624803508));
#6576=CARTESIAN_POINT('Ctrl Pts',(-25.6632984183101,0.965291239666668,2.3485275986422));
#6577=CARTESIAN_POINT('Ctrl Pts',(-25.6473893995262,0.960834612092796,2.35104651772394));
#6578=CARTESIAN_POINT('Ctrl Pts',(-25.6159251530686,0.951180080790835,2.35644914953997));
#6579=CARTESIAN_POINT('Ctrl Pts',(-25.6003693864663,0.945982332371016,2.35933277792001));
#6580=CARTESIAN_POINT('Ctrl Pts',(-25.5696010487147,0.934857849827407,2.36543410266168));
#6581=CARTESIAN_POINT('Ctrl Pts',(-25.554388497757,0.928931075544407,2.36865182569908));
#6582=CARTESIAN_POINT('Ctrl Pts',(-25.5092553225566,0.910065915709691,2.378761754307));
#6583=CARTESIAN_POINT('Ctrl Pts',(-25.4798364380125,0.896042727572782,2.3861116959914));
#6584=CARTESIAN_POINT('Ctrl Pts',(-25.4438909156586,0.876699211680765,2.39591502278523));
#6585=CARTESIAN_POINT('Ctrl Pts',(-25.4367414461902,0.872737300160877,2.39790741951298));
#6586=CARTESIAN_POINT('Ctrl Pts',(-25.4225293356803,0.864633016249678,2.40194902287731));
#6587=CARTESIAN_POINT('Ctrl Pts',(-25.4154580969326,0.860484766397168,2.40400099723935));
#6588=CARTESIAN_POINT('Ctrl Pts',(-25.3944657161042,0.847820800232131,2.41021024122678));
#6589=CARTESIAN_POINT('Ctrl Pts',(-25.380746070164,0.839077244133138,2.41442548123448));
#6590=CARTESIAN_POINT('Ctrl Pts',(-25.3538260232817,0.820989195886628,2.42297767676368));
#6591=CARTESIAN_POINT('Ctrl Pts',(-25.3406279393829,0.811646297981065,2.42731389565943));
#6592=CARTESIAN_POINT('Ctrl Pts',(-25.3147430597672,0.792367900936231,2.43607407349852));
#6593=CARTESIAN_POINT('Ctrl Pts',(-25.3020562810124,0.782432389835529,2.44049806007427));
#6594=CARTESIAN_POINT('Ctrl Pts',(-25.2771860341754,0.761968758341592,2.4494026816381));
#6595=CARTESIAN_POINT('Ctrl Pts',(-25.2650025732109,0.751440637442868,2.45388334271684));
#6596=CARTESIAN_POINT('Ctrl Pts',(-25.2411353303519,0.729786781206718,2.46287109582098));
#6597=CARTESIAN_POINT('Ctrl Pts',(-25.2294515461917,0.718661056693567,2.46737821378511));
#6598=CARTESIAN_POINT('Ctrl Pts',(-25.2065843288473,0.695801899103863,2.47638907712378));
#6599=CARTESIAN_POINT('Ctrl Pts',(-25.1954014188971,0.684068711345197,2.48089267439045));
#6600=CARTESIAN_POINT('Ctrl Pts',(-25.1790045373378,0.666000870018046,2.48762367211154));
#6601=CARTESIAN_POINT('Ctrl Pts',(-25.1735960376354,0.659892776183967,2.48986579326023));
#6602=CARTESIAN_POINT('Ctrl Pts',(-25.1629494208789,0.647568638488018,2.49431990834339));
#6603=CARTESIAN_POINT('Ctrl Pts',(-25.1577105174054,0.641352897528938,2.49653204883515));
#6604=CARTESIAN_POINT('Ctrl Pts',(-25.1319358378313,0.610000274169434,2.50751029184406));
#6605=CARTESIAN_POINT('Ctrl Pts',(-25.1126431635002,0.584053957250259,2.51603030353834));
#6606=CARTESIAN_POINT('Ctrl Pts',(-25.0766559633797,0.53042915613372,2.53234045288691));
#6607=CARTESIAN_POINT('Ctrl Pts',(-25.0599598863832,0.502751233364297,2.54013165293879));
#6608=CARTESIAN_POINT('Ctrl Pts',(-25.0368787132278,0.459895387665409,2.55112212486568));
#6609=CARTESIAN_POINT('Ctrl Pts',(-25.0295127265205,0.445386602515356,2.55466961647924));
#6610=CARTESIAN_POINT('Ctrl Pts',(-25.015447538885,0.415909836891662,2.56150652151535));
#6611=CARTESIAN_POINT('Ctrl Pts',(-25.0087479847154,0.400940313195683,2.56479614450175));
#6612=CARTESIAN_POINT('Ctrl Pts',(-24.9992124578344,0.378134446441368,2.56951620636084));
#6613=CARTESIAN_POINT('Ctrl Pts',(-24.9961153890925,0.370461653972984,2.57105596109368));
#6614=CARTESIAN_POINT('Ctrl Pts',(-24.9901146400105,0.35504609621479,2.57405082283814));
#6615=CARTESIAN_POINT('Ctrl Pts',(-24.9872162178828,0.347318031889454,2.57550327285404));
#6616=CARTESIAN_POINT('Ctrl Pts',(-24.978823527118,0.324069285671265,2.57972387330156));
#6617=CARTESIAN_POINT('Ctrl Pts',(-24.9736218334904,0.308462402151712,2.58236010535198));
#6618=CARTESIAN_POINT('Ctrl Pts',(-24.9640099750406,0.277069749192375,2.58725894187429));
#6619=CARTESIAN_POINT('Ctrl Pts',(-24.9595973255169,0.261278097086917,2.58952279476209));
#6620=CARTESIAN_POINT('Ctrl Pts',(-24.9515543557535,0.229504132582814,2.59366790173025));
#6621=CARTESIAN_POINT('Ctrl Pts',(-24.9479240403419,0.21352182008315,2.59554916744327));
#6622=CARTESIAN_POINT('Ctrl Pts',(-24.941447441202,0.181365268356563,2.59891718319404));
#6623=CARTESIAN_POINT('Ctrl Pts',(-24.9386011499407,0.165191031604556,2.60040394522677));
#6624=CARTESIAN_POINT('Ctrl Pts',(-24.9337002237304,0.132648091777223,2.60297035508353));
#6625=CARTESIAN_POINT('Ctrl Pts',(-24.93164556828,0.116279393924669,2.60405001587272));
#6626=CARTESIAN_POINT('Ctrl Pts',(-24.928341708171,0.0833436511207344,2.60578872210515));
#6627=CARTESIAN_POINT('Ctrl Pts',(-24.9270927815557,0.0667757724171855,
2.60644761593105));
#6628=CARTESIAN_POINT('Ctrl Pts',(-24.9258378814317,0.041773714006671,2.60711000800063));
#6629=CARTESIAN_POINT('Ctrl Pts',(-24.9255229363957,0.0334016706388515,
2.60727635262696));
#6630=CARTESIAN_POINT('Ctrl Pts',(-24.9251040599288,0.0166741935422472,
2.60749761997639));
#6631=CARTESIAN_POINT('Ctrl Pts',(-24.9249998216784,0.00832709294464485,
2.6075527040951));
#6632=CARTESIAN_POINT('Ctrl Pts',(-24.925,1.55854062294791E-16,2.60755260924175));
#6633=CARTESIAN_POINT('',(-27.0987792489536,-0.00011176064453429,2.99999999791826));
#6634=CARTESIAN_POINT('',(-24.7512207470268,-1.35620146123698E-16,3.));
#6635=CARTESIAN_POINT('Ctrl Pts',(-27.0987792489536,-0.000111760644534305,
2.99999999791826));
#6636=CARTESIAN_POINT('Ctrl Pts',(-27.098788175703,0.125293846590081,3.00000466972209));
#6637=CARTESIAN_POINT('Ctrl Pts',(-27.0836572608919,0.249887612487841,2.9920480612095));
#6638=CARTESIAN_POINT('Ctrl Pts',(-27.0242841101371,0.48924794879498,2.96225146824175));
#6639=CARTESIAN_POINT('Ctrl Pts',(-26.9807678619007,0.603149705374038,2.94076784698434));
#6640=CARTESIAN_POINT('Ctrl Pts',(-26.8427192011934,0.860536585807651,2.87814965124371));
#6641=CARTESIAN_POINT('Ctrl Pts',(-26.7376907200816,0.989566183851768,2.83419679721349));
#6642=CARTESIAN_POINT('Ctrl Pts',(-26.5155467319979,1.17588715226968,2.76143949975893));
#6643=CARTESIAN_POINT('Ctrl Pts',(-26.4004065512224,1.24404280001839,2.73036038773098));
#6644=CARTESIAN_POINT('Ctrl Pts',(-26.1626806024216,1.32927584783701,2.68979319984401));
#6645=CARTESIAN_POINT('Ctrl Pts',(-26.045246827223,1.35044153732405,2.67886312720281));
#6646=CARTESIAN_POINT('Ctrl Pts',(-25.8046235970333,1.35043417397338,2.67886683912841));
#6647=CARTESIAN_POINT('Ctrl Pts',(-25.6870707985615,1.32923939483604,2.68981328055148));
#6648=CARTESIAN_POINT('Ctrl Pts',(-25.449853763149,1.24407674422564,2.73034115324469));
#6649=CARTESIAN_POINT('Ctrl Pts',(-25.3353287651276,1.17639337787472,2.76120614485189));
#6650=CARTESIAN_POINT('Ctrl Pts',(-25.1094606312558,0.987455834851943,2.83506483214577));
#6651=CARTESIAN_POINT('Ctrl Pts',(-25.0061794065546,0.857630793528194,2.87869860737062));
#6652=CARTESIAN_POINT('Ctrl Pts',(-24.8702787932864,0.605712510755168,2.94025713869639));
#6653=CARTESIAN_POINT('Ctrl Pts',(-24.8263223973941,0.491220877838436,2.96195070021859));
#6654=CARTESIAN_POINT('Ctrl Pts',(-24.7664326588165,0.250724694262543,2.99199929730303));
#6655=CARTESIAN_POINT('Ctrl Pts',(-24.7512189476652,0.125688720919145,3.));
#6656=CARTESIAN_POINT('Ctrl Pts',(-24.7512207470268,-1.77808824465813E-16,
3.));
#6657=CARTESIAN_POINT('',(-26.9249999965755,-8.27588207139558E-5,2.60755260743233));
#6658=CARTESIAN_POINT('',(-27.0987792489536,-0.00011176064453429,2.99999999791826));
#6659=CARTESIAN_POINT('',(-26.925,-1.22464679914735E-16,2.60755336253159));
#6660=CARTESIAN_POINT('Ctrl Pts',(-26.9249999965755,-8.27588207141801E-5,
2.60755260743234));
#6661=CARTESIAN_POINT('Ctrl Pts',(-26.9249999988585,-5.51724988970155E-5,
2.60755260869231));
#6662=CARTESIAN_POINT('Ctrl Pts',(-26.925,-2.75862252988456E-5,2.60755260934744));
#6663=CARTESIAN_POINT('Ctrl Pts',(-26.925,-1.18762492463923E-16,2.60755260939777));
#6664=CARTESIAN_POINT('',(-24.925,7.79270311473956E-17,2.60755260924175));
#6665=CARTESIAN_POINT('Ctrl Pts',(-26.925,-1.18762492463923E-16,2.60755260939777));
#6666=CARTESIAN_POINT('Ctrl Pts',(-26.925,0.056804854575246,2.60755271302727));
#6667=CARTESIAN_POINT('Ctrl Pts',(-26.9201545072349,0.11340491023323,2.60497728285419));
#6668=CARTESIAN_POINT('Ctrl Pts',(-26.9010104955459,0.22498623920327,2.5949812948901));
#6669=CARTESIAN_POINT('Ctrl Pts',(-26.8867435237432,0.279664869028097,2.58757303140779));
#6670=CARTESIAN_POINT('Ctrl Pts',(-26.8304379456036,0.439261093144634,2.55919607531663));
#6671=CARTESIAN_POINT('Ctrl Pts',(-26.7755419497675,0.537393100961416,2.5323069913651));
#6672=CARTESIAN_POINT('Ctrl Pts',(-26.6644533472358,0.676591305065292,2.48451442941931));
#6673=CARTESIAN_POINT('Ctrl Pts',(-26.6171007671406,0.72494248878711,2.46539574358495));
#6674=CARTESIAN_POINT('Ctrl Pts',(-26.4737133682738,0.844473887402666,2.41369606443502));
#6675=CARTESIAN_POINT('Ctrl Pts',(-26.36820386171,0.904656958254169,2.38211334429286));
#6676=CARTESIAN_POINT('Ctrl Pts',(-26.1484453864065,0.980999063110147,2.34001084161921));
#6677=CARTESIAN_POINT('Ctrl Pts',(-26.0378922085563,1.00000218800714,2.32842180399996));
#6678=CARTESIAN_POINT('Ctrl Pts',(-25.8119011916325,0.999997808364593,2.32843245470472));
#6679=CARTESIAN_POINT('Ctrl Pts',(-25.7011902899078,0.980940359915184,2.3400492095282));
#6680=CARTESIAN_POINT('Ctrl Pts',(-25.4813838789149,0.904439026472466,2.38222657916133));
#6681=CARTESIAN_POINT('Ctrl Pts',(-25.3760142250183,0.844278486742472,2.41378709535218));
#6682=CARTESIAN_POINT('Ctrl Pts',(-25.1812462928254,0.681847452255209,2.48402790420268));
#6683=CARTESIAN_POINT('Ctrl Pts',(-25.095560456034,0.575048470588331,2.52290226852294));
#6684=CARTESIAN_POINT('Ctrl Pts',(-24.998457233114,0.384117255242701,2.56961701508285));
#6685=CARTESIAN_POINT('Ctrl Pts',(-24.9711794271723,0.310565523100897,2.58353335930288));
#6686=CARTESIAN_POINT('Ctrl Pts',(-24.9343517093779,0.15745257163897,2.60255728285402));
#6687=CARTESIAN_POINT('Ctrl Pts',(-24.925,0.0790612261660938,2.60754968635441));
#6688=CARTESIAN_POINT('Ctrl Pts',(-24.925,1.53956708492938E-16,2.60755260924175));
#6689=CARTESIAN_POINT('',(-24.7512207470268,-1.35620146123698E-16,3.));
#6690=CARTESIAN_POINT('Origin',(-28.425,0.,0.));
#6691=CARTESIAN_POINT('',(-21.125,-2.82842712474618,1.00000000000001));
#6692=CARTESIAN_POINT('',(-21.125,-2.82842712474618,-1.00000000000001));
#6693=CARTESIAN_POINT('Origin',(-21.125,1.33651518465759E-15,0.));
#6694=CARTESIAN_POINT('',(-28.425,-2.82842712474619,-1.00000000000001));
#6695=CARTESIAN_POINT('',(-28.425,-2.82842712474619,-1.00000000000001));
#6696=CARTESIAN_POINT('',(-28.425,2.82842712474619,-1.00000000000001));
#6697=CARTESIAN_POINT('Origin',(-28.425,1.00559551819496E-31,0.));
#6698=CARTESIAN_POINT('',(-21.125,2.82842712474619,-1.00000000000001));
#6699=CARTESIAN_POINT('',(-28.425,2.82842712474619,-1.00000000000001));
#6700=CARTESIAN_POINT('',(-21.125,3.,-3.67394039744206E-16));
#6701=CARTESIAN_POINT('Origin',(-21.125,1.33651518465759E-15,0.));
#6702=CARTESIAN_POINT('',(-20.325,3.,-3.67394039744206E-16));
#6703=CARTESIAN_POINT('',(-28.425,3.,-3.67394039744206E-16));
#6704=CARTESIAN_POINT('Origin',(-20.325,9.30296956444027E-16,0.));
#6705=CARTESIAN_POINT('',(-21.125,2.82842712474619,0.999999999999995));
#6706=CARTESIAN_POINT('Origin',(-21.125,1.33651518465759E-15,0.));
#6707=CARTESIAN_POINT('',(-28.425,2.82842712474619,1.00000000000001));
#6708=CARTESIAN_POINT('',(-28.425,2.82842712474619,1.00000000000001));
#6709=CARTESIAN_POINT('',(-28.425,-2.82842712474619,1.00000000000001));
#6710=CARTESIAN_POINT('Origin',(-28.425,1.00559551819496E-31,0.));
#6711=CARTESIAN_POINT('',(-28.425,-2.82842712474619,1.00000000000001));
#6712=CARTESIAN_POINT('Ctrl Pts',(-24.7512207470268,1.465751492483E-15,
-3.));
#6713=CARTESIAN_POINT('Ctrl Pts',(-24.7512225835704,0.128285957454602,-3.));
#6714=CARTESIAN_POINT('Ctrl Pts',(-24.7670495401009,0.25583672234664,-2.99166914509907));
#6715=CARTESIAN_POINT('Ctrl Pts',(-24.8294109793546,0.500872203914624,-2.96042265250318));
#6716=CARTESIAN_POINT('Ctrl Pts',(-24.8750650035884,0.617122189157838,-2.9379400782468));
#6717=CARTESIAN_POINT('Ctrl Pts',(-25.014086994418,0.868531543834054,-2.87533793314114));
#6718=CARTESIAN_POINT('Ctrl Pts',(-25.1178167867906,0.996326582468178,-2.83188528988297));
#6719=CARTESIAN_POINT('Ctrl Pts',(-25.343381297619,1.1815076728687,-2.75895840349069));
#6720=CARTESIAN_POINT('Ctrl Pts',(-25.4571148445719,1.24753580132896,-2.72873792314024));
#6721=CARTESIAN_POINT('Ctrl Pts',(-25.7218191299461,1.34070762403808,-2.68430500111959));
#6722=CARTESIAN_POINT('Ctrl Pts',(-25.8409376382471,1.35029210277812,-2.67893845828434));
#6723=CARTESIAN_POINT('Ctrl Pts',(-26.0070593989418,1.35058323368467,-2.67879169700489));
#6724=CARTESIAN_POINT('Ctrl Pts',(-26.1263048541123,1.34103185276652,-2.684134010337));
#6725=CARTESIAN_POINT('Ctrl Pts',(-26.391961880762,1.24815768478947,-2.72845580912919));
#6726=CARTESIAN_POINT('Ctrl Pts',(-26.5066389202574,1.18160031466836,-2.75893875380659));
#6727=CARTESIAN_POINT('Ctrl Pts',(-26.7321634254033,0.99620726980863,-2.83191131674452));
#6728=CARTESIAN_POINT('Ctrl Pts',(-26.8354958588566,0.868962163429233,-2.8751698727339));
#6729=CARTESIAN_POINT('Ctrl Pts',(-26.9742467036987,0.618608250844591,-2.93761533941595));
#6730=CARTESIAN_POINT('Ctrl Pts',(-27.0198972430111,0.502744502919277,-2.96008325572955));
#6731=CARTESIAN_POINT('Ctrl Pts',(-27.0826499193283,0.257871735999257,-2.99151091633777));
#6732=CARTESIAN_POINT('Ctrl Pts',(-27.0987700470889,0.129382268032874,-2.99999518213318));
#6733=CARTESIAN_POINT('Ctrl Pts',(-27.0987792489536,0.000111760644532495,
-2.99999999791826));
#6734=CARTESIAN_POINT('Ctrl Pts',(-24.7512207470268,-3.65455693999632E-16,
3.));
#6735=CARTESIAN_POINT('Ctrl Pts',(-24.7512225835705,-0.128285957454966,
3.));
#6736=CARTESIAN_POINT('Ctrl Pts',(-24.7670495401008,-0.255836722348032,
2.99166914509913));
#6737=CARTESIAN_POINT('Ctrl Pts',(-24.8294109793572,-0.500872203922864,
2.9604226525019));
#6738=CARTESIAN_POINT('Ctrl Pts',(-24.8750650035926,-0.617122189167466,
2.93794007824478));
#6739=CARTESIAN_POINT('Ctrl Pts',(-25.0140869944243,-0.868531543842818,
2.87533793313844));
#6740=CARTESIAN_POINT('Ctrl Pts',(-25.1178167867974,-0.996326582475323,
2.8318852898804));
#6741=CARTESIAN_POINT('Ctrl Pts',(-25.3433812976256,-1.18150767287279,2.75895840348889));
#6742=CARTESIAN_POINT('Ctrl Pts',(-25.4571148445771,-1.24753580133114,2.72873792313922));
#6743=CARTESIAN_POINT('Ctrl Pts',(-25.7218191299552,-1.34070762404087,2.68430500111824));
#6744=CARTESIAN_POINT('Ctrl Pts',(-25.8409376382588,-1.35029210277812,2.67893845828434));
#6745=CARTESIAN_POINT('Ctrl Pts',(-26.0070593989402,-1.35058323368466,2.67879169700489));
#6746=CARTESIAN_POINT('Ctrl Pts',(-26.12630485411,-1.34103185276689,2.6841340103368));
#6747=CARTESIAN_POINT('Ctrl Pts',(-26.3919618807593,-1.2481576847908,2.72845580912858));
#6748=CARTESIAN_POINT('Ctrl Pts',(-26.506638920255,-1.18160031466976,2.75893875380596));
#6749=CARTESIAN_POINT('Ctrl Pts',(-26.7321634253999,-0.996207269812109,
2.83191131674325));
#6750=CARTESIAN_POINT('Ctrl Pts',(-26.835495858853,-0.868962163433963,2.87516987273241));
#6751=CARTESIAN_POINT('Ctrl Pts',(-26.9742467036962,-0.618608250850395,
2.93761533941474));
#6752=CARTESIAN_POINT('Ctrl Pts',(-27.0198972430095,-0.502744502924232,
2.96008325572877));
#6753=CARTESIAN_POINT('Ctrl Pts',(-27.0826499193282,-0.257871736000858,
2.99151091633771));
#6754=CARTESIAN_POINT('Ctrl Pts',(-27.0987700470889,-0.129382268034096,
2.99999518213318));
#6755=CARTESIAN_POINT('Ctrl Pts',(-27.0987792489536,-0.000111760644534299,
2.99999999791826));
#6756=CARTESIAN_POINT('Origin',(-25.925,0.,-3.));
#6757=CARTESIAN_POINT('',(-26.925,-1.22464679914735E-16,-1.00000000000001));
#6758=CARTESIAN_POINT('',(-26.925,-1.22464679914735E-16,-3.));
#6759=CARTESIAN_POINT('Origin',(-25.925,0.,-1.00000000000001));
#6760=CARTESIAN_POINT('Ctrl Pts',(-26.9249999965755,8.27588207122151E-5,
-2.60755260743233));
#6761=CARTESIAN_POINT('Ctrl Pts',(-26.9249904249565,0.115739541719608,-2.60754732495302));
#6762=CARTESIAN_POINT('Ctrl Pts',(-26.9050186532092,0.229309368673701,-2.59676308014965));
#6763=CARTESIAN_POINT('Ctrl Pts',(-26.8283116849146,0.443793157962873,-2.55814777286124));
#6764=CARTESIAN_POINT('Ctrl Pts',(-26.7725502043353,0.542252124779991,-2.53089457930302));
#6765=CARTESIAN_POINT('Ctrl Pts',(-26.6216961833966,0.728812739977055,-2.46627281639632));
#6766=CARTESIAN_POINT('Ctrl Pts',(-26.5220865225859,0.812534660967263,-2.42818900421659));
#6767=CARTESIAN_POINT('Ctrl Pts',(-26.3104040242462,0.929588521928789,-2.36930439148383));
#6768=CARTESIAN_POINT('Ctrl Pts',(-26.2022893987898,0.967702137191157,-2.34728407052782));
#6769=CARTESIAN_POINT('Ctrl Pts',(-26.0338171724686,0.995597707881966,-2.33105492627662));
#6770=CARTESIAN_POINT('Ctrl Pts',(-25.9787262626432,1.00008101773999,-2.32837603269168));
#6771=CARTESIAN_POINT('Ctrl Pts',(-25.8686962905677,0.999917360916853,-2.32847915347898));
#6772=CARTESIAN_POINT('Ctrl Pts',(-25.8139981228262,0.995338596268691,-2.33120606433384));
#6773=CARTESIAN_POINT('Ctrl Pts',(-25.6457369572163,0.967153847373896,-2.34760035492249));
#6774=CARTESIAN_POINT('Ctrl Pts',(-25.537535323688,0.928753670996883,-2.36976707795452));
#6775=CARTESIAN_POINT('Ctrl Pts',(-25.3255406714156,0.810864803745833,-2.42897889523396));
#6776=CARTESIAN_POINT('Ctrl Pts',(-25.2257850797804,0.72648986790713,-2.46725895286466));
#6777=CARTESIAN_POINT('Ctrl Pts',(-25.0755270452445,0.539171378437474,-2.53180070351224));
#6778=CARTESIAN_POINT('Ctrl Pts',(-25.0202559439194,0.440786335108821,-2.55885563811918));
#6779=CARTESIAN_POINT('Ctrl Pts',(-24.9446246649158,0.227289219833161,-2.59695611074295));
#6780=CARTESIAN_POINT('Ctrl Pts',(-24.925,0.114639026798552,-2.60755684743726));
#6781=CARTESIAN_POINT('Ctrl Pts',(-24.925,2.65813431825893E-16,-2.60755260924174));
#6782=CARTESIAN_POINT('Origin',(-25.925,0.,-3.));
#6783=CARTESIAN_POINT('',(-26.925,-1.22464679914735E-16,1.));
#6784=CARTESIAN_POINT('Origin',(-25.925,0.,1.));
#6785=CARTESIAN_POINT('',(-26.925,-1.22464679914735E-16,-3.));
#6786=CARTESIAN_POINT('Ctrl Pts',(-26.9249999965755,-8.27588207141808E-5,
2.60755260743234));
#6787=CARTESIAN_POINT('Ctrl Pts',(-26.9249904249565,-0.115739541719426,
2.6075473249531));
#6788=CARTESIAN_POINT('Ctrl Pts',(-26.9050186532092,-0.229309368673756,
2.59676308014972));
#6789=CARTESIAN_POINT('Ctrl Pts',(-26.8283116849141,-0.443793157963809,
2.55814777286102));
#6790=CARTESIAN_POINT('Ctrl Pts',(-26.7725502043348,-0.542252124780864,
2.53089457930282));
#6791=CARTESIAN_POINT('Ctrl Pts',(-26.6216961833953,-0.728812739978349,
2.46627281639579));
#6792=CARTESIAN_POINT('Ctrl Pts',(-26.5220865225849,-0.81253466096794,2.42818900421627));
#6793=CARTESIAN_POINT('Ctrl Pts',(-26.3104040242456,-0.929588521929025,
2.36930439148371));
#6794=CARTESIAN_POINT('Ctrl Pts',(-26.202289398789,-0.967702137191383,2.3472840705277));
#6795=CARTESIAN_POINT('Ctrl Pts',(-26.0338171724679,-0.995597707882035,
2.33105492627659));
#6796=CARTESIAN_POINT('Ctrl Pts',(-25.9787262626427,-1.00008101774,2.32837603269168));
#6797=CARTESIAN_POINT('Ctrl Pts',(-25.8686962905678,-0.999917360916838,
2.32847915347901));
#6798=CARTESIAN_POINT('Ctrl Pts',(-25.8139981228264,-0.995338596268709,
2.33120606433384));
#6799=CARTESIAN_POINT('Ctrl Pts',(-25.6457369572167,-0.967153847373996,
2.34760035492244));
#6800=CARTESIAN_POINT('Ctrl Pts',(-25.5375353236883,-0.928753670997002,
2.36976707795446));
#6801=CARTESIAN_POINT('Ctrl Pts',(-25.3255406714161,-0.810864803746178,
2.42897889523381));
#6802=CARTESIAN_POINT('Ctrl Pts',(-25.2257850797809,-0.726489867907553,
2.46725895286448));
#6803=CARTESIAN_POINT('Ctrl Pts',(-25.0755270452453,-0.539171378438706,
2.53180070351187));
#6804=CARTESIAN_POINT('Ctrl Pts',(-25.0202559439199,-0.440786335109945,
2.558855638119));
#6805=CARTESIAN_POINT('Ctrl Pts',(-24.9446246649148,-0.227289219830435,
2.59695611074344));
#6806=CARTESIAN_POINT('Ctrl Pts',(-24.925,-0.114639026795822,2.60755684743755));
#6807=CARTESIAN_POINT('Ctrl Pts',(-24.925,6.24162981673305E-17,2.60755260924175));
#6808=CARTESIAN_POINT('Origin',(0.,0.,0.));
#6809=CARTESIAN_POINT('',(-19.525,-2.3,-2.81668763803891E-16));
#6810=CARTESIAN_POINT('Origin',(-19.525,8.93680102069846E-16,0.));
#6811=CARTESIAN_POINT('',(-20.325,-2.3,-2.81668763803891E-16));
#6812=CARTESIAN_POINT('',(-1.05273456325769E-16,-2.3,-2.81668763803891E-16));
#6813=CARTESIAN_POINT('Origin',(-20.325,9.30296956444027E-16,0.));
#6814=CARTESIAN_POINT('Origin',(28.225,1.03717240014867E-14,0.));
#6815=CARTESIAN_POINT('',(28.225,1.15,-1.40834381901944E-16));
#6816=CARTESIAN_POINT('Origin',(28.225,1.03717240014867E-14,0.));
#6817=CARTESIAN_POINT('',(28.425,0.949999999999984,-1.16341445918995E-16));
#6818=CARTESIAN_POINT('',(28.225,1.15,-1.40834381901944E-16));
#6819=CARTESIAN_POINT('Origin',(28.425,1.04083408558608E-14,0.));
#6820=CARTESIAN_POINT('Origin',(-28.425,0.,0.));
#6821=CARTESIAN_POINT('',(23.575,1.15,-1.40834381901944E-16));
#6822=CARTESIAN_POINT('Origin',(23.575,9.52038213728696E-15,0.));
#6823=CARTESIAN_POINT('',(-28.425,1.14999999999999,-1.40834381901944E-16));
#6824=CARTESIAN_POINT('Origin',(-28.425,0.,0.));
#6825=CARTESIAN_POINT('',(6.975,1.5,-1.83697019872102E-16));
#6826=CARTESIAN_POINT('Origin',(6.975,6.48118322422997E-15,0.));
#6827=CARTESIAN_POINT('',(23.575,1.5,-1.83697019872102E-16));
#6828=CARTESIAN_POINT('',(-28.425,1.49999999999999,-1.83697019872102E-16));
#6829=CARTESIAN_POINT('Origin',(23.575,9.52038213728696E-15,0.));
#6830=CARTESIAN_POINT('Origin',(6.975,6.48118322422997E-15,0.));
#6831=CARTESIAN_POINT('',(1.875,2.5,-3.06161699786838E-16));
#6832=CARTESIAN_POINT('Origin',(1.875,5.54745343768837E-15,0.));
#6833=CARTESIAN_POINT('',(6.975,2.,-2.4492935982947E-16));
#6834=CARTESIAN_POINT('',(6.975,2.,-2.4492935982947E-16));
#6835=CARTESIAN_POINT('Origin',(6.975,6.48118322422997E-15,0.));
#6836=CARTESIAN_POINT('Origin',(-28.425,0.,0.));
#6837=CARTESIAN_POINT('',(-19.525,3.,-3.67394039744206E-16));
#6838=CARTESIAN_POINT('Origin',(-19.525,8.93680102069846E-16,0.));
#6839=CARTESIAN_POINT('',(1.875,3.,-3.67394039744206E-16));
#6840=CARTESIAN_POINT('',(-28.425,3.,-3.67394039744206E-16));
#6841=CARTESIAN_POINT('Origin',(1.875,5.54745343768837E-15,0.));
#6842=CARTESIAN_POINT('Origin',(1.875,3.,0.));
#6843=CARTESIAN_POINT('Origin',(6.975,2.,0.));
#6844=CARTESIAN_POINT('Origin',(23.575,1.5,0.));
#6845=CARTESIAN_POINT('Origin',(28.425,1.15,0.));
#6846=CARTESIAN_POINT('Origin',(-20.325,-3.,0.));
#6847=CARTESIAN_POINT('Origin',(-19.525,-3.,0.));
#6848=CARTESIAN_POINT('Ctrl Pts',(-24.7512201965622,-1.76183904791747E-16,
3.00000124311957));
#6849=CARTESIAN_POINT('Ctrl Pts',(-24.7512206151827,-0.0224904615946165,
3.00000102486114));
#6850=CARTESIAN_POINT('Ctrl Pts',(-24.7517085809449,-0.0449131097845628,
2.99974818887592));
#6851=CARTESIAN_POINT('Ctrl Pts',(-24.7536439761057,-0.0895752885321344,
2.99874684907646));
#6852=CARTESIAN_POINT('Ctrl Pts',(-24.7550910425168,-0.111823263408201,
2.99799854559508));
#6853=CARTESIAN_POINT('Ctrl Pts',(-24.7608541223484,-0.1783210198246,2.99502561769244));
#6854=CARTESIAN_POINT('Ctrl Pts',(-24.7665915611397,-0.222335311776171,
2.99207181620778));
#6855=CARTESIAN_POINT('Ctrl Pts',(-24.7780288192454,-0.287837360410401,
2.98624162780084));
#6856=CARTESIAN_POINT('Ctrl Pts',(-24.7823197307722,-0.309606561385091,
2.9840619482597));
#6857=CARTESIAN_POINT('Ctrl Pts',(-24.7894679779366,-0.342109798413635,
2.98045092915735));
#6858=CARTESIAN_POINT('Ctrl Pts',(-24.7919724393738,-0.352930055186467,
2.97918882741414));
#6859=CARTESIAN_POINT('Ctrl Pts',(-24.7972214032702,-0.374523340751585,
2.97655141398561));
#6860=CARTESIAN_POINT('Ctrl Pts',(-24.7999681707864,-0.385302896814476,
2.97517498996412));
#6861=CARTESIAN_POINT('Ctrl Pts',(-24.8085247289755,-0.417396325006835,
2.97090101111401));
#6862=CARTESIAN_POINT('Ctrl Pts',(-24.8146611612218,-0.438519664833829,
2.96785340267611));
#6863=CARTESIAN_POINT('Ctrl Pts',(-24.827780795185,-0.480245605735743,2.96138777142348));
#6864=CARTESIAN_POINT('Ctrl Pts',(-24.8347634091537,-0.500846985261598,
2.95797002138279));
#6865=CARTESIAN_POINT('Ctrl Pts',(-24.8569585745012,-0.561885306302581,
2.94720211826449));
#6866=CARTESIAN_POINT('Ctrl Pts',(-24.8734157851973,-0.601558415893414,
2.93933707448591));
#6867=CARTESIAN_POINT('Ctrl Pts',(-24.9005699650057,-0.659577946472712,
2.92666307786021));
#6868=CARTESIAN_POINT('Ctrl Pts',(-24.9100343005407,-0.678670330222981,
2.92229185258577));
#6869=CARTESIAN_POINT('Ctrl Pts',(-24.9297925040438,-0.71635605219561,2.91328291034591));
#6870=CARTESIAN_POINT('Ctrl Pts',(-24.9400941970776,-0.734962854491018,
2.90864166879988));
#6871=CARTESIAN_POINT('Ctrl Pts',(-24.9615143509208,-0.771630108002665,
2.8991297911222));
#6872=CARTESIAN_POINT('Ctrl Pts',(-24.9725542617936,-0.789558390564698,
2.89429401664935));
#6873=CARTESIAN_POINT('Ctrl Pts',(-24.9953081681755,-0.824675412874891,
2.88448450367961));
#6874=CARTESIAN_POINT('Ctrl Pts',(-25.0070176561689,-0.841856330313478,
2.87951274183948));
#6875=CARTESIAN_POINT('Ctrl Pts',(-25.0431332882325,-0.892293349065707,
2.86444629839692));
#6876=CARTESIAN_POINT('Ctrl Pts',(-25.0685240643679,-0.92444624815415,2.85419987571196));
#6877=CARTESIAN_POINT('Ctrl Pts',(-25.1085917532924,-0.970519332950307,
2.83872559859403));
#6878=CARTESIAN_POINT('Ctrl Pts',(-25.1222785365167,-0.985516952511357,
2.83355000263622));
#6879=CARTESIAN_POINT('Ctrl Pts',(-25.1503245087481,-1.0147915600932,2.82319808714425));
#6880=CARTESIAN_POINT('Ctrl Pts',(-25.1646905450052,-1.02907433729268,2.81801945772866));
#6881=CARTESIAN_POINT('Ctrl Pts',(-25.1940839460452,-1.05688985201168,2.80770598732435));
#6882=CARTESIAN_POINT('Ctrl Pts',(-25.2091788350748,-1.07047868451993,2.80254912945966));
#6883=CARTESIAN_POINT('Ctrl Pts',(-25.2397857985023,-1.09666875082295,2.79240445901191));
#6884=CARTESIAN_POINT('Ctrl Pts',(-25.255320223101,-1.10929658351522,2.78740768552752));
#6885=CARTESIAN_POINT('Ctrl Pts',(-25.2868469170525,-1.13362940492584,2.77760057560582));
#6886=CARTESIAN_POINT('Ctrl Pts',(-25.302839623016,-1.14533536930589,2.77278994432858));
#6887=CARTESIAN_POINT('Ctrl Pts',(-25.3352860491081,-1.16783592991971,2.76338858760642));
#6888=CARTESIAN_POINT('Ctrl Pts',(-25.3517397751987,-1.17863049873125,2.75879782839759));
#6889=CARTESIAN_POINT('Ctrl Pts',(-25.4018014264425,-1.20964993058026,2.74540766718039));
#6890=CARTESIAN_POINT('Ctrl Pts',(-25.4361157965431,-1.22851722530086,2.7369879943305));
#6891=CARTESIAN_POINT('Ctrl Pts',(-25.4890319606085,-1.25402748115622,2.72534609489846));
#6892=CARTESIAN_POINT('Ctrl Pts',(-25.5069294362475,-1.26207118462111,2.72162720547797));
#6893=CARTESIAN_POINT('Ctrl Pts',(-25.5341341065867,-1.27341479768989,2.71632858891394));
#6894=CARTESIAN_POINT('Ctrl Pts',(-25.5432727036745,-1.27707929627404,2.71460725980808));
#6895=CARTESIAN_POINT('Ctrl Pts',(-25.5616696134459,-1.28416319515221,2.71126336921716));
#6896=CARTESIAN_POINT('Ctrl Pts',(-25.5709426986925,-1.28758734347613,2.70963852456332));
#6897=CARTESIAN_POINT('Ctrl Pts',(-25.5987920948568,-1.29743244195315,2.70494558321287));
#6898=CARTESIAN_POINT('Ctrl Pts',(-25.617433882299,-1.30344363716717,2.70205116137013));
#6899=CARTESIAN_POINT('Ctrl Pts',(-25.6548879621502,-1.31438372733535,2.69674641877482));
#6900=CARTESIAN_POINT('Ctrl Pts',(-25.6736968490448,-1.31931173160548,2.69433651551851));
#6901=CARTESIAN_POINT('Ctrl Pts',(-25.7303690237763,-1.33248274213305,2.68786059982172));
#6902=CARTESIAN_POINT('Ctrl Pts',(-25.7684773832559,-1.33911643529056,2.6845486252675));
#6903=CARTESIAN_POINT('Ctrl Pts',(-25.8261391213393,-1.34582410918546,2.68118864483476));
#6904=CARTESIAN_POINT('Ctrl Pts',(-25.8454430068625,-1.34751862690545,2.68033657178926));
#6905=CARTESIAN_POINT('Ctrl Pts',(-25.8842203794928,-1.34980853567155,2.67918411053143));
#6906=CARTESIAN_POINT('Ctrl Pts',(-25.9037051371427,-1.35040321450496,2.67888411665589));
#6907=CARTESIAN_POINT('Ctrl Pts',(-25.9428031440834,-1.35047173299045,2.67884957398269));
#6908=CARTESIAN_POINT('Ctrl Pts',(-25.9625262788923,-1.34993763378488,2.67911903945913));
#6909=CARTESIAN_POINT('Ctrl Pts',(-26.001675179068,-1.34774256849848,2.68022395142751));
#6910=CARTESIAN_POINT('Ctrl Pts',(-26.0211401464231,-1.34608753889995,2.68105638390197));
#6911=CARTESIAN_POINT('Ctrl Pts',(-26.0598521561959,-1.34168374443805,2.68326288816889));
#6912=CARTESIAN_POINT('Ctrl Pts',(-26.0790999491839,-1.33893558390626,2.68463664029074));
#6913=CARTESIAN_POINT('Ctrl Pts',(-26.1173832731121,-1.33236285214624,2.68790468740719));
#6914=CARTESIAN_POINT('Ctrl Pts',(-26.1364187960914,-1.3285382337657,2.6897989878991));
#6915=CARTESIAN_POINT('Ctrl Pts',(-26.1932112333693,-1.31546132541517,2.69623160867151));
#6916=CARTESIAN_POINT('Ctrl Pts',(-26.230658868257,-1.30460568802834,2.70152164206104));
#6917=CARTESIAN_POINT('Ctrl Pts',(-26.2769394358952,-1.28835579481113,2.70927322407079));
#6918=CARTESIAN_POINT('Ctrl Pts',(-26.2861736873588,-1.28496804550343,2.71088197061785));
#6919=CARTESIAN_POINT('Ctrl Pts',(-26.3045801226384,-1.27792632816734,2.71420859259991));
#6920=CARTESIAN_POINT('Ctrl Pts',(-26.3137696612827,-1.27426435838069,2.71593014837302));
#6921=CARTESIAN_POINT('Ctrl Pts',(-26.3411343470425,-1.26292005406289,2.72123342520569));
#6922=CARTESIAN_POINT('Ctrl Pts',(-26.3591086288947,-1.25488236548527,2.72495256846718));
#6923=CARTESIAN_POINT('Ctrl Pts',(-26.3945730991822,-1.23786441433935,2.73272536195925));
#6924=CARTESIAN_POINT('Ctrl Pts',(-26.4120574252086,-1.22888679609906,2.73677778918298));
#6925=CARTESIAN_POINT('Ctrl Pts',(-26.4465443911629,-1.21000870437874,2.74517655409933));
#6926=CARTESIAN_POINT('Ctrl Pts',(-26.4635470144595,-1.20010820517651,2.74952291627504));
#6927=CARTESIAN_POINT('Ctrl Pts',(-26.4970806133762,-1.17939058963319,2.75847308374743));
#6928=CARTESIAN_POINT('Ctrl Pts',(-26.5136115807888,-1.16857346524795,2.76307691198199));
#6929=CARTESIAN_POINT('Ctrl Pts',(-26.5462080833809,-1.14602103189425,2.77250675337683));
#6930=CARTESIAN_POINT('Ctrl Pts',(-26.5622736983626,-1.1342856634169,2.77733281570969));
#6931=CARTESIAN_POINT('Ctrl Pts',(-26.5939416429695,-1.10988763337467,2.78717256703881));
#6932=CARTESIAN_POINT('Ctrl Pts',(-26.609547564207,-1.09722193187051,2.79218745199254));
#6933=CARTESIAN_POINT('Ctrl Pts',(-26.6402813438902,-1.07095721724289,2.8023664037371));
#6934=CARTESIAN_POINT('Ctrl Pts',(-26.655295080658,-1.05745634546246,2.80749236059604));
#6935=CARTESIAN_POINT('Ctrl Pts',(-26.6846548548111,-1.02971401041123,2.81778570291711));
#6936=CARTESIAN_POINT('Ctrl Pts',(-26.698997953854,-1.01547501212971,2.82295214467571));
#6937=CARTESIAN_POINT('Ctrl Pts',(-26.7270253212179,-0.9862662210335,2.83328911051859));
#6938=CARTESIAN_POINT('Ctrl Pts',(-26.7407095447861,-0.971296396677904,
2.83845969056953));
#6939=CARTESIAN_POINT('Ctrl Pts',(-26.7807872610901,-0.925288863725475,
2.85392633511737));
#6940=CARTESIAN_POINT('Ctrl Pts',(-26.8062107356642,-0.893151941339901,
2.864178670324));
#6941=CARTESIAN_POINT('Ctrl Pts',(-26.8423947744529,-0.842704579251605,
2.87926472137709));
#6942=CARTESIAN_POINT('Ctrl Pts',(-26.8541358893937,-0.825504953419079,
2.88424727122285));
#6943=CARTESIAN_POINT('Ctrl Pts',(-26.8712465648999,-0.799139107619217,
2.89162033090013));
#6944=CARTESIAN_POINT('Ctrl Pts',(-26.8768710845513,-0.790248327529814,
2.89406322620423));
#6945=CARTESIAN_POINT('Ctrl Pts',(-26.8879472162261,-0.772282090199619,
2.89890928529195));
#6946=CARTESIAN_POINT('Ctrl Pts',(-26.8934095805383,-0.763187949365317,
2.9013172405501));
#6947=CARTESIAN_POINT('Ctrl Pts',(-26.9094752397211,-0.735724969537462,
2.90844874441802));
#6948=CARTESIAN_POINT('Ctrl Pts',(-26.9197553059395,-0.717185246436077,
2.91307852354811));
#6949=CARTESIAN_POINT('Ctrl Pts',(-26.939491662068,-0.679606241243712,2.92207399934037));
#6950=CARTESIAN_POINT('Ctrl Pts',(-26.9489441843561,-0.660573675186057,
2.92643805302077));
#6951=CARTESIAN_POINT('Ctrl Pts',(-26.9760664924627,-0.602745972669873,
2.93909208245404));
#6952=CARTESIAN_POINT('Ctrl Pts',(-26.9925039932974,-0.563222492320479,
2.94694446393472));
#6953=CARTESIAN_POINT('Ctrl Pts',(-27.0220719282814,-0.482184935663518,
2.96128319208414));
#6954=CARTESIAN_POINT('Ctrl Pts',(-27.0352038812473,-0.440658278132651,
2.96777086803717));
#6955=CARTESIAN_POINT('Ctrl Pts',(-27.0523220500515,-0.376834051179656,
2.97631783456127));
#6956=CARTESIAN_POINT('Ctrl Pts',(-27.0576008937577,-0.355274612711083,
2.97897112077082));
#6957=CARTESIAN_POINT('Ctrl Pts',(-27.0672604256937,-0.311662928430509,
2.98384906046174));
#6958=CARTESIAN_POINT('Ctrl Pts',(-27.0716118507556,-0.28974195783202,2.98605887165636));
#6959=CARTESIAN_POINT('Ctrl Pts',(-27.0793664061891,-0.245626216202856,
2.99001098961276));
#6960=CARTESIAN_POINT('Ctrl Pts',(-27.0827665013565,-0.223449220869781,
2.99175175446374));
#6961=CARTESIAN_POINT('Ctrl Pts',(-27.0886129441394,-0.178789236716059,
2.99475258363014));
#6962=CARTESIAN_POINT('Ctrl Pts',(-27.0910452438611,-0.15640475955994,2.99600543335325));
#6963=CARTESIAN_POINT('Ctrl Pts',(-27.0968540554839,-0.089380072836346,
2.99900191231137));
#6964=CARTESIAN_POINT('Ctrl Pts',(-27.0987766251388,-0.0447217917816824,
2.99999958185766));
#6965=CARTESIAN_POINT('Ctrl Pts',(-27.0987813865579,0.02219325478624,3.00000207062791));
#6966=CARTESIAN_POINT('Ctrl Pts',(-27.098302980501,0.0444882044529776,2.99975417679133));
#6967=CARTESIAN_POINT('Ctrl Pts',(-27.0963851499708,0.0890579606384697,
2.99876191230976));
#6968=CARTESIAN_POINT('Ctrl Pts',(-27.0949457527391,0.111332767632207,2.99801754221172));
#6969=CARTESIAN_POINT('Ctrl Pts',(-27.091097912228,0.155862099946067,2.99603257401337));
#6970=CARTESIAN_POINT('Ctrl Pts',(-27.0886882785475,0.178121325914285,2.99479136150237));
#6971=CARTESIAN_POINT('Ctrl Pts',(-27.0828893311938,0.222600421497831,2.99181469259339));
#6972=CARTESIAN_POINT('Ctrl Pts',(-27.0794844211542,0.244888534479486,2.99007132802239));
#6973=CARTESIAN_POINT('Ctrl Pts',(-27.0717763207677,0.288870061738483,2.98614250919086));
#6974=CARTESIAN_POINT('Ctrl Pts',(-27.0674611935747,0.310670506014752,2.98395091125391));
#6975=CARTESIAN_POINT('Ctrl Pts',(-27.0579367437935,0.353839565051259,2.9791402804281));
#6976=CARTESIAN_POINT('Ctrl Pts',(-27.0527261874502,0.375218601036114,2.97652060572815));
#6977=CARTESIAN_POINT('Ctrl Pts',(-27.0357699204893,0.438751951157216,2.96805162738344));
#6978=CARTESIAN_POINT('Ctrl Pts',(-27.022699391642,0.480310643319706,2.9615908339538));
#6979=CARTESIAN_POINT('Ctrl Pts',(-27.0004758229384,0.541446694763495,2.95080875849622));
#6980=CARTESIAN_POINT('Ctrl Pts',(-26.992623681753,0.561640072316629,2.94702942050088));
#6981=CARTESIAN_POINT('Ctrl Pts',(-26.9801909795193,0.591614335345463,2.94110596088858));
#6982=CARTESIAN_POINT('Ctrl Pts',(-26.9759332605878,0.60156226518298,2.9390870305072));
#6983=CARTESIAN_POINT('Ctrl Pts',(-26.9671990237161,0.621350626541985,2.9349673711246));
#6984=CARTESIAN_POINT('Ctrl Pts',(-26.9627163520765,0.631203409825238,2.93286380405279));
#6985=CARTESIAN_POINT('Ctrl Pts',(-26.9490003388169,0.660466615132205,2.92646369421333));
#6986=CARTESIAN_POINT('Ctrl Pts',(-26.9394866261483,0.679617007741926,2.92207164107701));
#6987=CARTESIAN_POINT('Ctrl Pts',(-26.9197263731453,0.717239156030636,2.91306539958487));
#6988=CARTESIAN_POINT('Ctrl Pts',(-26.9094813066202,0.735708225799572,2.9084518514383));
#6989=CARTESIAN_POINT('Ctrl Pts',(-26.8776651907974,0.790114397662365,2.89432752559281));
#6990=CARTESIAN_POINT('Ctrl Pts',(-26.855015951808,0.825052668578728,2.88453262436396));
#6991=CARTESIAN_POINT('Ctrl Pts',(-26.8188828130475,0.875511458559016,2.86945918682943));
#6992=CARTESIAN_POINT('Ctrl Pts',(-26.806477865951,0.892005672721574,2.86437109863276));
#6993=CARTESIAN_POINT('Ctrl Pts',(-26.7809370903558,0.924343794681297,2.85409960048903));
#6994=CARTESIAN_POINT('Ctrl Pts',(-26.7678062754663,0.94018178468473,2.84891809889914));
#6995=CARTESIAN_POINT('Ctrl Pts',(-26.747534952965,0.963465362975877,2.8410930742898));
#6996=CARTESIAN_POINT('Ctrl Pts',(-26.7406847515848,0.971143336910766,2.83847720905191));
#6997=CARTESIAN_POINT('Ctrl Pts',(-26.726866828362,0.986257778221377,2.8332609577602));
#6998=CARTESIAN_POINT('Ctrl Pts',(-26.7198864405152,0.993708965489587,2.83065565931379));
#6999=CARTESIAN_POINT('Ctrl Pts',(-26.6987545667654,1.01572267126073,2.82286342050641));
#7000=CARTESIAN_POINT('Ctrl Pts',(-26.6843929425923,1.02996804274084,2.81769254606288));
#7001=CARTESIAN_POINT('Ctrl Pts',(-26.6405196961263,1.07140451601384,2.80231490014364));
#7002=CARTESIAN_POINT('Ctrl Pts',(-26.6101990167324,1.09732522138671,2.79223355729096));
#7003=CARTESIAN_POINT('Ctrl Pts',(-26.5630920876351,1.13367314163991,2.77758248050925));
#7004=CARTESIAN_POINT('Ctrl Pts',(-26.5471176954077,1.14536678978723,2.77277705423988));
#7005=CARTESIAN_POINT('Ctrl Pts',(-26.5146128603087,1.16790420277309,2.76335982199196));
#7006=CARTESIAN_POINT('Ctrl Pts',(-26.4980824626504,1.17874802188457,2.75874796251914));
#7007=CARTESIAN_POINT('Ctrl Pts',(-26.4644489769846,1.19957326674856,2.74975657993441));
#7008=CARTESIAN_POINT('Ctrl Pts',(-26.4473526605441,1.20955077156384,2.74537877233407));
#7009=CARTESIAN_POINT('Ctrl Pts',(-26.4212418428209,1.22386659438305,2.73901196687352));
#7010=CARTESIAN_POINT('Ctrl Pts',(-26.4124621517901,1.228528090482,2.73692383614117));
#7011=CARTESIAN_POINT('Ctrl Pts',(-26.3948579023758,1.23757356026446,2.73284557774276));
#7012=CARTESIAN_POINT('Ctrl Pts',(-26.3860148872854,1.24196849424176,2.73085066873684));
#7013=CARTESIAN_POINT('Ctrl Pts',(-26.341645261955,1.26327266721299,2.72112112107028));
#7014=CARTESIAN_POINT('Ctrl Pts',(-26.3055755853367,1.27824593843012,2.71409299783002));
#7015=CARTESIAN_POINT('Ctrl Pts',(-26.2323061069552,1.30408058177653,2.70177489330743));
#7016=CARTESIAN_POINT('Ctrl Pts',(-26.1951017095151,1.31494712049099,2.69648267860914));
#7017=CARTESIAN_POINT('Ctrl Pts',(-26.1384101250037,1.32811617463851,2.69000746444321));
#7018=CARTESIAN_POINT('Ctrl Pts',(-26.1193652332726,1.33198320784822,2.68809291154564));
#7019=CARTESIAN_POINT('Ctrl Pts',(-26.0809718851876,1.3386498031086,2.68477922262698));
#7020=CARTESIAN_POINT('Ctrl Pts',(-26.0616267484912,1.34144867007465,2.68338047067986));
#7021=CARTESIAN_POINT('Ctrl Pts',(-26.032363761062,1.34482540214699,2.68168886075706));
#7022=CARTESIAN_POINT('Ctrl Pts',(-26.0225572765905,1.34581398544558,2.6811927471385));
#7023=CARTESIAN_POINT('Ctrl Pts',(-26.0029866880182,1.34750220702749,2.68034468497323));
#7024=CARTESIAN_POINT('Ctrl Pts',(-25.9932072525691,1.34820413161832,2.67999159504196));
#7025=CARTESIAN_POINT('Ctrl Pts',(-25.9639248763077,1.34988314454028,2.6791465090366));
#7026=CARTESIAN_POINT('Ctrl Pts',(-25.944430256616,1.35043954651561,2.67886577671177));
#7027=CARTESIAN_POINT('Ctrl Pts',(-25.8861245439706,1.3504378095549,2.67886672345498));
#7028=CARTESIAN_POINT('Ctrl Pts',(-25.8474103812661,1.34822168461923,2.67998726078285));
#7029=CARTESIAN_POINT('Ctrl Pts',(-25.7896108997839,1.34161043104656,2.68329952853649));
#7030=CARTESIAN_POINT('Ctrl Pts',(-25.77038745646,1.33885814096473,2.68467529043326));
#7031=CARTESIAN_POINT('Ctrl Pts',(-25.7320267290187,1.33225068682402,2.68796030874541));
#7032=CARTESIAN_POINT('Ctrl Pts',(-25.7128830247106,1.32839365293775,2.68987049972103));
#7033=CARTESIAN_POINT('Ctrl Pts',(-25.684251748041,1.32177623227189,2.69312505274073));
#7034=CARTESIAN_POINT('Ctrl Pts',(-25.6747141290368,1.31942923189441,2.69427597594583));
#7035=CARTESIAN_POINT('Ctrl Pts',(-25.6556602502347,1.31445363734784,2.69670691417443));
#7036=CARTESIAN_POINT('Ctrl Pts',(-25.6461499439873,1.31182592199724,2.69798646989669));
#7037=CARTESIAN_POINT('Ctrl Pts',(-25.6178199688841,1.30356690507148,2.70199177974632));
#7038=CARTESIAN_POINT('Ctrl Pts',(-25.5991462839436,1.29754850153216,2.7048898077093));
#7039=CARTESIAN_POINT('Ctrl Pts',(-25.5622141869212,1.28451064624858,2.71110556040655));
#7040=CARTESIAN_POINT('Ctrl Pts',(-25.5439551422566,1.27749140423903,2.71442318809091));
#7041=CARTESIAN_POINT('Ctrl Pts',(-25.5078398888184,1.26246846951838,2.7214427902055));
#7042=CARTESIAN_POINT('Ctrl Pts',(-25.4899837037464,1.25446472257528,2.72514479532609));
#7043=CARTESIAN_POINT('Ctrl Pts',(-25.4370072942282,1.22898847560418,2.73677631458511));
#7044=CARTESIAN_POINT('Ctrl Pts',(-25.4024760017176,1.21005101589909,2.74523245622064));
#7045=CARTESIAN_POINT('Ctrl Pts',(-25.3602838735484,1.18392877826526,2.75651122868636));
#7046=CARTESIAN_POINT('Ctrl Pts',(-25.3518919706823,1.17857845856369,2.75880349026457));
#7047=CARTESIAN_POINT('Ctrl Pts',(-25.3352100824015,1.16763411776591,2.76345337348231));
#7048=CARTESIAN_POINT('Ctrl Pts',(-25.3269100051743,1.16203215951806,2.76581417940247));
#7049=CARTESIAN_POINT('Ctrl Pts',(-25.3022695725318,1.14493024612509,2.77295794310452));
#7050=CARTESIAN_POINT('Ctrl Pts',(-25.2861657292169,1.13312260725419,2.77780759607733));
#7051=CARTESIAN_POINT('Ctrl Pts',(-25.2545675218788,1.10869580205534,2.78764693628012));
#7052=CARTESIAN_POINT('Ctrl Pts',(-25.2390758775543,1.09607878865392,2.7926357760188));
#7053=CARTESIAN_POINT('Ctrl Pts',(-25.208692728647,1.07004449005284,2.80271440082356));
#7054=CARTESIAN_POINT('Ctrl Pts',(-25.193801243974,1.05662718870003,2.80780421768086));
#7055=CARTESIAN_POINT('Ctrl Pts',(-25.1646090505302,1.02899230331321,2.81804902565378));
#7056=CARTESIAN_POINT('Ctrl Pts',(-25.150308350114,1.0147747185966,2.82320404678685));
#7057=CARTESIAN_POINT('Ctrl Pts',(-25.1222934624824,0.985532507337768,2.83354449797841));
#7058=CARTESIAN_POINT('Ctrl Pts',(-25.1085792726074,0.970507895413088,2.83872995787953));
#7059=CARTESIAN_POINT('Ctrl Pts',(-25.0817381947277,0.939637998238792,2.84909699750195));
#7060=CARTESIAN_POINT('Ctrl Pts',(-25.0686119208846,0.923793044275968,2.8542784068245));
#7061=CARTESIAN_POINT('Ctrl Pts',(-25.0493655924709,0.89939352728851,2.86202245059147));
#7062=CARTESIAN_POINT('Ctrl Pts',(-25.0430172047533,0.891144919357543,2.86460202126226));
#7063=CARTESIAN_POINT('Ctrl Pts',(-25.0305204210295,0.874501923571608,2.86972650110557));
#7064=CARTESIAN_POINT('Ctrl Pts',(-25.02437110194,0.866107944767956,2.87227157889308));
#7065=CARTESIAN_POINT('Ctrl Pts',(-24.9941173036171,0.823768140450452,2.88490209785398));
#7066=CARTESIAN_POINT('Ctrl Pts',(-24.971471952131,0.788729223015757,2.89470441040782));
#7067=CARTESIAN_POINT('Ctrl Pts',(-24.9292309034491,0.716312201964233,2.91346931208067));
#7068=CARTESIAN_POINT('Ctrl Pts',(-24.9096333854723,0.67893485651281,2.92243312349527));
#7069=CARTESIAN_POINT('Ctrl Pts',(-24.882541170584,0.621060652496465,2.93507771188247));
#7070=CARTESIAN_POINT('Ctrl Pts',(-24.8738951241542,0.601467423657377,2.93915911726366));
#7071=CARTESIAN_POINT('Ctrl Pts',(-24.8573856909762,0.561660850722054,2.94702500788258));
#7072=CARTESIAN_POINT('Ctrl Pts',(-24.8495218895994,0.541445422596672,2.95080973422482));
#7073=CARTESIAN_POINT('Ctrl Pts',(-24.8383292807319,0.510647491444322,2.95624018705409));
#7074=CARTESIAN_POINT('Ctrl Pts',(-24.8346940039926,0.500285853504753,2.95801168194031));
#7075=CARTESIAN_POINT('Ctrl Pts',(-24.8276504459147,0.47946808360172,2.96145728412088));
#7076=CARTESIAN_POINT('Ctrl Pts',(-24.8242483365591,0.469031804392166,2.96312833452968));
#7077=CARTESIAN_POINT('Ctrl Pts',(-24.8143971656437,0.43763579155551,2.96798415471264));
#7078=CARTESIAN_POINT('Ctrl Pts',(-24.8082915227193,0.416559647886907,2.97101715178475));
#7079=CARTESIAN_POINT('Ctrl Pts',(-24.7970093173975,0.374165786036183,2.97665328568467));
#7080=CARTESIAN_POINT('Ctrl Pts',(-24.7918298385069,0.352840123671072,2.97925785882102));
#7081=CARTESIAN_POINT('Ctrl Pts',(-24.782389163039,0.309931323851521,2.98402682340998));
#7082=CARTESIAN_POINT('Ctrl Pts',(-24.7781279721287,0.288348186260506,2.98619122824603));
#7083=CARTESIAN_POINT('Ctrl Pts',(-24.7705258708633,0.244922725747236,2.99006614582328));
#7084=CARTESIAN_POINT('Ctrl Pts',(-24.7671849516661,0.223080406167033,2.99177667236476));
#7085=CARTESIAN_POINT('Ctrl Pts',(-24.7614323434624,0.179133152105929,2.99472933868235));
#7086=CARTESIAN_POINT('Ctrl Pts',(-24.7590206303916,0.157028224677869,2.99597149337493));
#7087=CARTESIAN_POINT('Ctrl Pts',(-24.7551426261223,0.112550514170608,2.99797188287434));
#7088=CARTESIAN_POINT('Ctrl Pts',(-24.7536766612853,0.0901766051585178,
2.99872994324477));
#7089=CARTESIAN_POINT('Ctrl Pts',(-24.7522036848644,0.056412851214161,2.99949202836053));
#7090=CARTESIAN_POINT('Ctrl Pts',(-24.7518340087419,0.045106917611639,2.9996834086165));
#7091=CARTESIAN_POINT('Ctrl Pts',(-24.751342340005,0.0225174807118006,2.99993797771742));
#7092=CARTESIAN_POINT('Ctrl Pts',(-24.751219987252,0.0112452307973078,3.00000135224878));
#7093=CARTESIAN_POINT('Ctrl Pts',(-24.7512201965622,-1.76183904791747E-16,
3.00000124311957));
#7094=CARTESIAN_POINT('Ctrl Pts',(-24.925001560524,1.55857043960029E-16,
2.60754908509522));
#7095=CARTESIAN_POINT('Ctrl Pts',(-24.9250019171665,-0.0166541334801613,
2.60754889538878));
#7096=CARTESIAN_POINT('Ctrl Pts',(-24.9254176382407,-0.0332580512905814,
2.60732913473253));
#7097=CARTESIAN_POINT('Ctrl Pts',(-24.9270664927659,-0.0663302887433916,
2.60645878753386));
#7098=CARTESIAN_POINT('Ctrl Pts',(-24.9282993169708,-0.0828048613803104,
2.60580837511734));
#7099=CARTESIAN_POINT('Ctrl Pts',(-24.9332091568075,-0.132046292319869,
2.6032243577104));
#7100=CARTESIAN_POINT('Ctrl Pts',(-24.9380971518304,-0.164638771132326,
2.60065696465499));
#7101=CARTESIAN_POINT('Ctrl Pts',(-24.9478410920693,-0.2131428828209,2.59558946593898));
#7102=CARTESIAN_POINT('Ctrl Pts',(-24.9514967222119,-0.229262924518058,
2.59369492625983));
#7103=CARTESIAN_POINT('Ctrl Pts',(-24.957586651506,-0.253331494462499,2.59055629104135));
#7104=CARTESIAN_POINT('Ctrl Pts',(-24.9597203204629,-0.261343868943599,
2.58945929408072));
#7105=CARTESIAN_POINT('Ctrl Pts',(-24.9641921606581,-0.277333645699326,
2.58716690003975));
#7106=CARTESIAN_POINT('Ctrl Pts',(-24.9665322616052,-0.285315881401586,
2.58597053613621));
#7107=CARTESIAN_POINT('Ctrl Pts',(-24.9738219975603,-0.309080988873579,
2.58225566779538));
#7108=CARTESIAN_POINT('Ctrl Pts',(-24.9790499139481,-0.324722771924263,
2.57960673936175));
#7109=CARTESIAN_POINT('Ctrl Pts',(-24.9902271496198,-0.355620732215222,
2.57398692473798));
#7110=CARTESIAN_POINT('Ctrl Pts',(-24.9961759681728,-0.370876004900204,
2.57101627563854));
#7111=CARTESIAN_POINT('Ctrl Pts',(-25.015085077571,-0.416074736889795,2.5616570008748));
#7112=CARTESIAN_POINT('Ctrl Pts',(-25.0291057524579,-0.445452580460472,
2.55482084113838));
#7113=CARTESIAN_POINT('Ctrl Pts',(-25.0522396804357,-0.488415905271011,
2.54380482293415));
#7114=CARTESIAN_POINT('Ctrl Pts',(-25.060302794776,-0.502553770162814,2.54000542968693));
#7115=CARTESIAN_POINT('Ctrl Pts',(-25.0771357413066,-0.530459957917378,
2.53217501323324));
#7116=CARTESIAN_POINT('Ctrl Pts',(-25.0859122400396,-0.54423825089383,2.5281409265225));
#7117=CARTESIAN_POINT('Ctrl Pts',(-25.1041610805409,-0.571390265168159,
2.51987336730303));
#7118=CARTESIAN_POINT('Ctrl Pts',(-25.113566501909,-0.584666115891092,2.51567019594392));
#7119=CARTESIAN_POINT('Ctrl Pts',(-25.1329516291768,-0.610670187636849,
2.50714393728714));
#7120=CARTESIAN_POINT('Ctrl Pts',(-25.1429274949106,-0.623392616257929,
2.50282256806535));
#7121=CARTESIAN_POINT('Ctrl Pts',(-25.1736961072169,-0.660741109040536,
2.48972707655347));
#7122=CARTESIAN_POINT('Ctrl Pts',(-25.195327708338,-0.68455025456915,2.48082106354484));
#7123=CARTESIAN_POINT('Ctrl Pts',(-25.2294632644966,-0.718667264605278,
2.46737109007097));
#7124=CARTESIAN_POINT('Ctrl Pts',(-25.2411236814041,-0.729772966325544,
2.46287255176686));
#7125=CARTESIAN_POINT('Ctrl Pts',(-25.2650173694561,-0.751450743819418,
2.45387484623857));
#7126=CARTESIAN_POINT('Ctrl Pts',(-25.2772564740961,-0.762027106466302,
2.44937367130548));
#7127=CARTESIAN_POINT('Ctrl Pts',(-25.3022981003744,-0.782624429154989,
2.44040938158115));
#7128=CARTESIAN_POINT('Ctrl Pts',(-25.3151581491073,-0.792686927403681,
2.43592713010271));
#7129=CARTESIAN_POINT('Ctrl Pts',(-25.3412336664868,-0.81208060939496,2.42710955837504));
#7130=CARTESIAN_POINT('Ctrl Pts',(-25.3544681763255,-0.821431489558622,
2.42276644946543));
#7131=CARTESIAN_POINT('Ctrl Pts',(-25.3813272555676,-0.839449886111459,
2.41424227949637));
#7132=CARTESIAN_POINT('Ctrl Pts',(-25.3949521969405,-0.848118124975917,
2.41006096216709));
#7133=CARTESIAN_POINT('Ctrl Pts',(-25.4225948394221,-0.864779736753649,
2.40188946584663));
#7134=CARTESIAN_POINT('Ctrl Pts',(-25.4366125456109,-0.872773089361171,
2.39789925750829));
#7135=CARTESIAN_POINT('Ctrl Pts',(-25.4792624301743,-0.895742905086398,
2.38626076145437));
#7136=CARTESIAN_POINT('Ctrl Pts',(-25.5084964623614,-0.909714092086863,
2.37894252774089));
#7137=CARTESIAN_POINT('Ctrl Pts',(-25.5535782411859,-0.928604376053514,
2.36882359052986));
#7138=CARTESIAN_POINT('Ctrl Pts',(-25.5688259457879,-0.934560719395051,
2.36559119630036));
#7139=CARTESIAN_POINT('Ctrl Pts',(-25.5920028890314,-0.942960637972592,
2.36098573061775));
#7140=CARTESIAN_POINT('Ctrl Pts',(-25.599788491408,-0.945674190484402,2.35948958119256));
#7141=CARTESIAN_POINT('Ctrl Pts',(-25.6154616875292,-0.950919800805243,
2.35658312944661));
#7142=CARTESIAN_POINT('Ctrl Pts',(-25.6233618667185,-0.95345537451926,2.35517084263494));
#7143=CARTESIAN_POINT('Ctrl Pts',(-25.6470880823364,-0.960745646595251,
2.35109181935035));
#7144=CARTESIAN_POINT('Ctrl Pts',(-25.6629699013087,-0.965196922396583,
2.3485760380501));
#7145=CARTESIAN_POINT('Ctrl Pts',(-25.6948788004851,-0.973298033223291,
2.34396524772702));
#7146=CARTESIAN_POINT('Ctrl Pts',(-25.7109029793721,-0.976947208699515,
2.34187060158446));
#7147=CARTESIAN_POINT('Ctrl Pts',(-25.7591846810364,-0.98670031076137,2.33624184790048));
#7148=CARTESIAN_POINT('Ctrl Pts',(-25.7916509919276,-0.991612544814396,
2.33336313702002));
#7149=CARTESIAN_POINT('Ctrl Pts',(-25.8407757493374,-0.996579561426912,
2.33044270026262));
#7150=CARTESIAN_POINT('Ctrl Pts',(-25.8572216409297,-0.997834347780394,
2.32970209313936));
#7151=CARTESIAN_POINT('Ctrl Pts',(-25.8902579157094,-0.999530019791506,
2.32870039378829));
#7152=CARTESIAN_POINT('Ctrl Pts',(-25.9068579008084,-0.999970378057432,
2.32843964431104));
#7153=CARTESIAN_POINT('Ctrl Pts',(-25.940167339092,-1.00002111583351,2.3284096204183));
#7154=CARTESIAN_POINT('Ctrl Pts',(-25.9569704089505,-0.999625616638187,
2.32864383514006));
#7155=CARTESIAN_POINT('Ctrl Pts',(-25.9903232055858,-0.998000175999123,
2.32960420547288));
#7156=CARTESIAN_POINT('Ctrl Pts',(-26.0069063303974,-0.996774630505924,
2.33032774135208));
#7157=CARTESIAN_POINT('Ctrl Pts',(-26.0398869194724,-0.993513631149867,
2.33224559661821));
#7158=CARTESIAN_POINT('Ctrl Pts',(-26.056285023184,-0.991478624792919,2.33343963815292));
#7159=CARTESIAN_POINT('Ctrl Pts',(-26.0889003945458,-0.986611532510906,
2.33628016806539));
#7160=CARTESIAN_POINT('Ctrl Pts',(-26.105117655415,-0.983779411669397,2.33792666122145));
#7161=CARTESIAN_POINT('Ctrl Pts',(-26.1535018144212,-0.974095992046507,
2.34351778370753));
#7162=CARTESIAN_POINT('Ctrl Pts',(-26.1854052228443,-0.966057418299631,
2.34811578904634));
#7163=CARTESIAN_POINT('Ctrl Pts',(-26.2248338237297,-0.954024410911544,
2.35485332977763));
#7164=CARTESIAN_POINT('Ctrl Pts',(-26.2327009185887,-0.951515790581753,
2.35625162439446));
#7165=CARTESIAN_POINT('Ctrl Pts',(-26.2483822299402,-0.946301415592757,
2.35914306656481));
#7166=CARTESIAN_POINT('Ctrl Pts',(-26.2562112318338,-0.943589735649563,
2.36063941300517));
#7167=CARTESIAN_POINT('Ctrl Pts',(-26.2795244997708,-0.935189305203641,
2.36524892931282));
#7168=CARTESIAN_POINT('Ctrl Pts',(-26.2948376392117,-0.929237415872055,
2.36848154417623));
#7169=CARTESIAN_POINT('Ctrl Pts',(-26.325051496053,-0.916635663404123,2.37523752156304));
#7170=CARTESIAN_POINT('Ctrl Pts',(-26.3399472189906,-0.90998775838627,2.37875982107005));
#7171=CARTESIAN_POINT('Ctrl Pts',(-26.3693282937335,-0.896008576234018,
2.3860598819696));
#7172=CARTESIAN_POINT('Ctrl Pts',(-26.3838136313699,-0.888677280052333,
2.38983766464245));
#7173=CARTESIAN_POINT('Ctrl Pts',(-26.4123824877163,-0.873335934871314,
2.39761699508693));
#7174=CARTESIAN_POINT('Ctrl Pts',(-26.426465999434,-0.865325879915252,2.40161856279578));
#7175=CARTESIAN_POINT('Ctrl Pts',(-26.4542364991725,-0.848625856496643,
2.40981481750003));
#7176=CARTESIAN_POINT('Ctrl Pts',(-26.4679235551807,-0.839935843967816,
2.41400954723539));
#7177=CARTESIAN_POINT('Ctrl Pts',(-26.4949029725259,-0.821869160578,2.42256208855009));
#7178=CARTESIAN_POINT('Ctrl Pts',(-26.508198393727,-0.812490238648981,2.42692093963487));
#7179=CARTESIAN_POINT('Ctrl Pts',(-26.5343819518632,-0.79304127975015,2.43576830807167));
#7180=CARTESIAN_POINT('Ctrl Pts',(-26.5471728631521,-0.783043916212123,
2.44022370093141));
#7181=CARTESIAN_POINT('Ctrl Pts',(-26.5721858410977,-0.762500782893491,
2.4491704956747));
#7182=CARTESIAN_POINT('Ctrl Pts',(-26.5844054044419,-0.751956838431768,
2.45366107730754));
#7183=CARTESIAN_POINT('Ctrl Pts',(-26.6082832421287,-0.730327797889394,
2.46264578885994));
#7184=CARTESIAN_POINT('Ctrl Pts',(-26.6199414783443,-0.719242678452863,
2.46713996742474));
#7185=CARTESIAN_POINT('Ctrl Pts',(-26.654085577301,-0.68517420940159,2.48058330680097));
#7186=CARTESIAN_POINT('Ctrl Pts',(-26.6757450357663,-0.661376894583312,
2.48949445887105));
#7187=CARTESIAN_POINT('Ctrl Pts',(-26.7065719269914,-0.624020742585236,
2.50260699297805));
#7188=CARTESIAN_POINT('Ctrl Pts',(-26.7165747372153,-0.611284460442826,
2.50693773894737));
#7189=CARTESIAN_POINT('Ctrl Pts',(-26.7311521296313,-0.591760614150655,
2.51334627463049));
#7190=CARTESIAN_POINT('Ctrl Pts',(-26.7359439235075,-0.585177012577659,
2.51546959688903));
#7191=CARTESIAN_POINT('Ctrl Pts',(-26.7453802030872,-0.57187305643892,2.51968170745714));
#7192=CARTESIAN_POINT('Ctrl Pts',(-26.7500338491731,-0.565138866716563,
2.52177466043333));
#7193=CARTESIAN_POINT('Ctrl Pts',(-26.7637209428383,-0.54480259527845,2.52797323999352));
#7194=CARTESIAN_POINT('Ctrl Pts',(-26.7724790166661,-0.53107397428613,2.53199736377097));
#7195=CARTESIAN_POINT('Ctrl Pts',(-26.7892933503868,-0.503246810054303,
2.53981607542183));
#7196=CARTESIAN_POINT('Ctrl Pts',(-26.7973464004641,-0.489153240022056,
2.54360923524378));
#7197=CARTESIAN_POINT('Ctrl Pts',(-26.8204531754342,-0.446331963437201,
2.55460789831045));
#7198=CARTESIAN_POINT('Ctrl Pts',(-26.8344570585593,-0.417064919965779,
2.56143305219685));
#7199=CARTESIAN_POINT('Ctrl Pts',(-26.8596473785478,-0.357056801425746,
2.57389602618921));
#7200=CARTESIAN_POINT('Ctrl Pts',(-26.8708351093533,-0.326306410018251,
2.5795350016813));
#7201=CARTESIAN_POINT('Ctrl Pts',(-26.8854188856716,-0.279044721282975,
2.58696387685385));
#7202=CARTESIAN_POINT('Ctrl Pts',(-26.889916181885,-0.263080008230857,2.58927006723958));
#7203=CARTESIAN_POINT('Ctrl Pts',(-26.8981455932565,-0.23078565943978,2.59350988787545));
#7204=CARTESIAN_POINT('Ctrl Pts',(-26.9018527777375,-0.214553232694009,
2.5954306174658));
#7205=CARTESIAN_POINT('Ctrl Pts',(-26.9084592496751,-0.181885630631591,
2.59886572989619));
#7206=CARTESIAN_POINT('Ctrl Pts',(-26.9113559512979,-0.165463618176975,
2.60037877253407));
#7207=CARTESIAN_POINT('Ctrl Pts',(-26.9163368119689,-0.13239300581574,2.60298704123573));
#7208=CARTESIAN_POINT('Ctrl Pts',(-26.9184090029522,-0.115817353571131,
2.6040759965005));
#7209=CARTESIAN_POINT('Ctrl Pts',(-26.9233578038635,-0.0661857319676012,
2.60668048407777));
#7210=CARTESIAN_POINT('Ctrl Pts',(-26.9249957317331,-0.0331163807650857,
2.60754764115516));
#7211=CARTESIAN_POINT('Ctrl Pts',(-26.9249997882108,0.0164340525421226,
2.60754980435113));
#7212=CARTESIAN_POINT('Ctrl Pts',(-26.924592211501,0.0329434099001457,2.60733433932482));
#7213=CARTESIAN_POINT('Ctrl Pts',(-26.922958321114,0.0659472086648965,2.60647188023517));
#7214=CARTESIAN_POINT('Ctrl Pts',(-26.9217320306451,0.0824416504222714,
2.60582488664723));
#7215=CARTESIAN_POINT('Ctrl Pts',(-26.9184538736218,0.11541551540594,2.60409958669229));
#7216=CARTESIAN_POINT('Ctrl Pts',(-26.9164009929087,0.131898419449027,2.60302074629033));
#7217=CARTESIAN_POINT('Ctrl Pts',(-26.911460595836,0.164835084256703,2.60043347726538));
#7218=CARTESIAN_POINT('Ctrl Pts',(-26.9085597921968,0.181339379062666,2.59891817499628));
#7219=CARTESIAN_POINT('Ctrl Pts',(-26.9019928975065,0.213907595706393,2.59550331376099));
#7220=CARTESIAN_POINT('Ctrl Pts',(-26.8983166368945,0.230050772994289,2.59359841481876));
#7221=CARTESIAN_POINT('Ctrl Pts',(-26.8902023083891,0.262017358841772,2.58941709788185));
#7222=CARTESIAN_POINT('Ctrl Pts',(-26.8857631894022,0.277848484290424,2.58714012203647));
#7223=CARTESIAN_POINT('Ctrl Pts',(-26.8713173449163,0.324894779397641,2.57977903284149));
#7224=CARTESIAN_POINT('Ctrl Pts',(-26.8601819442124,0.355668892391147,2.57416342317006));
#7225=CARTESIAN_POINT('Ctrl Pts',(-26.8412486366545,0.400939993511194,2.56479183005488));
#7226=CARTESIAN_POINT('Ctrl Pts',(-26.8345590268073,0.415893141702933,2.56150689497222));
#7227=CARTESIAN_POINT('Ctrl Pts',(-26.823967020712,0.438089012396727,2.55635832654132));
#7228=CARTESIAN_POINT('Ctrl Pts',(-26.8203396689083,0.445455430851153,2.55460350724556));
#7229=CARTESIAN_POINT('Ctrl Pts',(-26.8128985600938,0.460108665512343,2.55102277071131));
#7230=CARTESIAN_POINT('Ctrl Pts',(-26.8090795604559,0.467404628169107,2.54919438667112));
#7231=CARTESIAN_POINT('Ctrl Pts',(-26.797394241101,0.489073962305602,2.54363152212406));
#7232=CARTESIAN_POINT('Ctrl Pts',(-26.789289060049,0.503254782620711,2.53981402566018));
#7233=CARTESIAN_POINT('Ctrl Pts',(-26.7724543674525,0.531113894213035,2.53198595664959));
#7234=CARTESIAN_POINT('Ctrl Pts',(-26.7637261115164,0.544790196579881,2.52797594056181));
#7235=CARTESIAN_POINT('Ctrl Pts',(-26.7366204601151,0.585077837829156,2.51569932133656));
#7236=CARTESIAN_POINT('Ctrl Pts',(-26.7173245039422,0.610949544590526,2.50718576295211));
#7237=CARTESIAN_POINT('Ctrl Pts',(-26.6865409768543,0.648314158915958,2.49408419229669));
#7238=CARTESIAN_POINT('Ctrl Pts',(-26.6759726166714,0.660528085389509,2.48966171422195));
#7239=CARTESIAN_POINT('Ctrl Pts',(-26.6542132239272,0.684474388015626,2.48073390605899));
#7240=CARTESIAN_POINT('Ctrl Pts',(-26.6430264626965,0.696202382055636,2.4762302346818));
#7241=CARTESIAN_POINT('Ctrl Pts',(-26.6257563658622,0.713443816566611,2.46942885891313));
#7242=CARTESIAN_POINT('Ctrl Pts',(-26.6199203558455,0.71912933805822,2.46715519418601));
#7243=CARTESIAN_POINT('Ctrl Pts',(-26.6081482145809,0.730321546007037,2.46262131897029));
#7244=CARTESIAN_POINT('Ctrl Pts',(-26.6022012925659,0.735839132509788,2.46035683871519));
#7245=CARTESIAN_POINT('Ctrl Pts',(-26.5841980514885,0.752140229430916,2.45358395979733));
#7246=CARTESIAN_POINT('Ctrl Pts',(-26.5719627057113,0.762688893231257,2.44908952535157));
#7247=CARTESIAN_POINT('Ctrl Pts',(-26.5345850153881,0.793372503429236,2.43572354204093));
#7248=CARTESIAN_POINT('Ctrl Pts',(-26.5087533968938,0.812566724291233,2.42696101356095));
#7249=CARTESIAN_POINT('Ctrl Pts',(-26.4686207796459,0.83948227304429,2.41422655155215));
#7250=CARTESIAN_POINT('Ctrl Pts',(-26.4550114406092,0.848141391767837,2.4100497583254));
#7251=CARTESIAN_POINT('Ctrl Pts',(-26.4273190367366,0.864830292639679,2.40186446327311));
#7252=CARTESIAN_POINT('Ctrl Pts',(-26.4132360104195,0.872860114977211,2.39785591495116));
#7253=CARTESIAN_POINT('Ctrl Pts',(-26.384582055835,0.888281159414966,2.39004076104537));
#7254=CARTESIAN_POINT('Ctrl Pts',(-26.3700168965852,0.895669478070531,2.38623564655444));
#7255=CARTESIAN_POINT('Ctrl Pts',(-26.3477718580352,0.906270310920229,2.38070172959633));
#7256=CARTESIAN_POINT('Ctrl Pts',(-26.3402920246762,0.909722137727452,2.3788867625548));
#7257=CARTESIAN_POINT('Ctrl Pts',(-26.3252941333419,0.916420286651386,2.37534201103856));
#7258=CARTESIAN_POINT('Ctrl Pts',(-26.3177603512233,0.919674724840875,2.37360807070524));
#7259=CARTESIAN_POINT('Ctrl Pts',(-26.2799597723219,0.935450414400031,2.36515131650747));
#7260=CARTESIAN_POINT('Ctrl Pts',(-26.2492303116149,0.946538086235351,2.35904259359383));
#7261=CARTESIAN_POINT('Ctrl Pts',(-26.1868085832625,0.965668578368483,2.34833591063874));
#7262=CARTESIAN_POINT('Ctrl Pts',(-26.1551124003162,0.973715224519582,2.34373600934578));
#7263=CARTESIAN_POINT('Ctrl Pts',(-26.1068141625445,0.983466877886528,2.33810786542034));
#7264=CARTESIAN_POINT('Ctrl Pts',(-26.0905889199931,0.986330406808494,2.33644376922427));
#7265=CARTESIAN_POINT('Ctrl Pts',(-26.0578798138568,0.991267004789931,2.33356356824836));
#7266=CARTESIAN_POINT('Ctrl Pts',(-26.0413987784432,0.993339559141257,2.33234779729884));
#7267=CARTESIAN_POINT('Ctrl Pts',(-26.0164682576784,0.995840021233325,2.33087747927257));
#7268=CARTESIAN_POINT('Ctrl Pts',(-26.0081136505026,0.996572064821657,2.33044626591382));
#7269=CARTESIAN_POINT('Ctrl Pts',(-25.9914405419907,0.997822188899716,2.3297091449783));
#7270=CARTESIAN_POINT('Ctrl Pts',(-25.983108979154,0.99834196239474,2.32940224532968));
#7271=CARTESIAN_POINT('Ctrl Pts',(-25.9581619401288,0.999585267481797,2.32866771122069));
#7272=CARTESIAN_POINT('Ctrl Pts',(-25.9415535530913,0.999997281825182,2.32842370354953));
#7273=CARTESIAN_POINT('Ctrl Pts',(-25.8918801633427,0.999995995609899,2.32842452644233));
#7274=CARTESIAN_POINT('Ctrl Pts',(-25.8588977400795,0.998354960350003,2.32939847806693));
#7275=CARTESIAN_POINT('Ctrl Pts',(-25.809655632564,0.993459342757429,2.3322774437906));
#7276=CARTESIAN_POINT('Ctrl Pts',(-25.7932782734797,0.991421278478362,2.33347323218692));
#7277=CARTESIAN_POINT('Ctrl Pts',(-25.7605969584102,0.986528474355782,2.33632851316856));
#7278=CARTESIAN_POINT('Ctrl Pts',(-25.7442875327586,0.983672349909096,2.33798881805762));
#7279=CARTESIAN_POINT('Ctrl Pts',(-25.7198951962202,0.978772165598707,2.34081761913493));
#7280=CARTESIAN_POINT('Ctrl Pts',(-25.7117696482312,0.977034217384609,2.34181798163729));
#7281=CARTESIAN_POINT('Ctrl Pts',(-25.6955367491711,0.973349801421764,2.34393091101302));
#7282=CARTESIAN_POINT('Ctrl Pts',(-25.6874344702097,0.971403984435815,2.34504307866984));
#7283=CARTESIAN_POINT('Ctrl Pts',(-25.6632988267017,0.96528820198757,2.34852442457186));
#7284=CARTESIAN_POINT('Ctrl Pts',(-25.6473898327442,0.960831588438278,2.35104334024925));
#7285=CARTESIAN_POINT('Ctrl Pts',(-25.6159256353873,0.951177087518203,2.35644596476354));
#7286=CARTESIAN_POINT('Ctrl Pts',(-25.6003698930602,0.945979355455201,2.35932958924631));
#7287=CARTESIAN_POINT('Ctrl Pts',(-25.5696016033233,0.934854907919272,2.36543090574196));
#7288=CARTESIAN_POINT('Ctrl Pts',(-25.5543890761051,0.928928152287264,2.36864862443055));
#7289=CARTESIAN_POINT('Ctrl Pts',(-25.5092559713361,0.910063051819399,2.37875853937475));
#7290=CARTESIAN_POINT('Ctrl Pts',(-25.4798371327009,0.896039907812121,2.38610847112559));
#7291=CARTESIAN_POINT('Ctrl Pts',(-25.4438916664408,0.876696452792296,2.39591178467007));
#7292=CARTESIAN_POINT('Ctrl Pts',(-25.4367422081294,0.872734553740163,2.39790417870507));
#7293=CARTESIAN_POINT('Ctrl Pts',(-25.4225301197978,0.86463029533237,2.40194577660712));
#7294=CARTESIAN_POINT('Ctrl Pts',(-25.415458892085,0.860482058534005,2.40399774819588));
#7295=CARTESIAN_POINT('Ctrl Pts',(-25.3944665440157,0.847818132221257,2.41020698379142));
#7296=CARTESIAN_POINT('Ctrl Pts',(-25.3807469194853,0.839074603637398,2.41442221810216));
#7297=CARTESIAN_POINT('Ctrl Pts',(-25.3538269146123,0.820986612312243,2.42297440207294));
#7298=CARTESIAN_POINT('Ctrl Pts',(-25.3406288513095,0.811643743807886,2.42731061510823));
#7299=CARTESIAN_POINT('Ctrl Pts',(-25.3147440120878,0.792365407430321,2.43607078110781));
#7300=CARTESIAN_POINT('Ctrl Pts',(-25.302057253131,0.782429927595721,2.44049476170448));
#7301=CARTESIAN_POINT('Ctrl Pts',(-25.2771870451046,0.761966360498873,2.44939937123357));
#7302=CARTESIAN_POINT('Ctrl Pts',(-25.2650036031527,0.751438272731137,2.45388002625663));
#7303=CARTESIAN_POINT('Ctrl Pts',(-25.2411363975391,0.729784484637599,2.46286776721369));
#7304=CARTESIAN_POINT('Ctrl Pts',(-25.2294526316117,0.718658795136038,2.46737487908639));
#7305=CARTESIAN_POINT('Ctrl Pts',(-25.2065854499521,0.695799709481914,2.47638573024673));
#7306=CARTESIAN_POINT('Ctrl Pts',(-25.1954025574532,0.684066558646466,2.48088932142673));
#7307=CARTESIAN_POINT('Ctrl Pts',(-25.1790057014816,0.665998774177082,2.48762031005077));
#7308=CARTESIAN_POINT('Ctrl Pts',(-25.1735972102193,0.659890699564589,2.4898624281692));
#7309=CARTESIAN_POINT('Ctrl Pts',(-25.162950610077,0.647566600651522,2.49431653723255));
#7310=CARTESIAN_POINT('Ctrl Pts',(-25.157711714779,0.641350879252783,2.49652867473457));
#7311=CARTESIAN_POINT('Ctrl Pts',(-25.1319370754269,0.609998354556983,2.50750690290623));
#7312=CARTESIAN_POINT('Ctrl Pts',(-25.1126444312025,0.584052119288382,2.51602690308558));
#7313=CARTESIAN_POINT('Ctrl Pts',(-25.0766572872409,0.530427486923958,2.53233703039074));
#7314=CARTESIAN_POINT('Ctrl Pts',(-25.059961236299,0.502749651254307,2.54012821991269));
#7315=CARTESIAN_POINT('Ctrl Pts',(-25.0368800991623,0.459893940418662,2.5511186769858));
#7316=CARTESIAN_POINT('Ctrl Pts',(-25.0295141239499,0.445385200926366,2.55466616380487));
#7317=CARTESIAN_POINT('Ctrl Pts',(-25.0154489582634,0.415908528063232,2.5615030596008));
#7318=CARTESIAN_POINT('Ctrl Pts',(-25.0087494145486,0.40093905147491,2.56479267814122));
#7319=CARTESIAN_POINT('Ctrl Pts',(-24.9992139025481,0.378133256488474,2.56951273362108));
#7320=CARTESIAN_POINT('Ctrl Pts',(-24.9961168386391,0.370460488165633,2.57105248627292));
#7321=CARTESIAN_POINT('Ctrl Pts',(-24.9901160989215,0.355044978918723,2.57404734396978));
#7322=CARTESIAN_POINT('Ctrl Pts',(-24.9872176813169,0.347316938912865,2.57549979202267));
#7323=CARTESIAN_POINT('Ctrl Pts',(-24.978825003649,0.324068265856255,2.57972038676598));
#7324=CARTESIAN_POINT('Ctrl Pts',(-24.9736233181388,0.30846143145007,2.5823566152535));
#7325=CARTESIAN_POINT('Ctrl Pts',(-24.9640114746886,0.277068877280406,2.58725544515496));
#7326=CARTESIAN_POINT('Ctrl Pts',(-24.9595988320509,0.261277274869764,2.58951929498313));
#7327=CARTESIAN_POINT('Ctrl Pts',(-24.9515558748388,0.229503410355285,2.59366439634911));
#7328=CARTESIAN_POINT('Ctrl Pts',(-24.9479255650923,0.213521148150428,2.59554565951957));
#7329=CARTESIAN_POINT('Ctrl Pts',(-24.9414489760593,0.181364697617431,2.59891367071842));
#7330=CARTESIAN_POINT('Ctrl Pts',(-24.9386026892397,0.165190511764198,2.60040043074176));
#7331=CARTESIAN_POINT('Ctrl Pts',(-24.9337017706775,0.13264767434638,2.60296683712999));
#7332=CARTESIAN_POINT('Ctrl Pts',(-24.9316471184334,0.116279028004551,2.60404649646));
#7333=CARTESIAN_POINT('Ctrl Pts',(-24.9283432634801,0.0833433888462451,
2.60578520034254));
#7334=CARTESIAN_POINT('Ctrl Pts',(-24.9270943388138,0.0667755622802239,
2.60644409327794));
#7335=CARTESIAN_POINT('Ctrl Pts',(-24.9258394406481,0.0417735825487931,
2.60710648445228));
#7336=CARTESIAN_POINT('Ctrl Pts',(-24.9255244961035,0.0334015655269924,
2.6072728288538));
#7337=CARTESIAN_POINT('Ctrl Pts',(-24.9251056202904,0.0166741410701568,
2.60749409590418));
#7338=CARTESIAN_POINT('Ctrl Pts',(-24.9250013822027,0.00832706674008074,
2.60754917994844));
#7339=CARTESIAN_POINT('Ctrl Pts',(-24.925001560524,1.55857043960029E-16,
2.60754908509522));
#7340=CARTESIAN_POINT('Ctrl Pts',(-24.7512201965622,1.27647978108407E-15,
-3.00000124311957));
#7341=CARTESIAN_POINT('Ctrl Pts',(-24.7512206151827,0.0224904615946214,
-3.00000102486114));
#7342=CARTESIAN_POINT('Ctrl Pts',(-24.7517085809449,0.0449131097845636,
-2.99974818887592));
#7343=CARTESIAN_POINT('Ctrl Pts',(-24.7536439761057,0.0895752885321371,
-2.99874684907646));
#7344=CARTESIAN_POINT('Ctrl Pts',(-24.7550910425168,0.111823263408203,-2.99799854559508));
#7345=CARTESIAN_POINT('Ctrl Pts',(-24.7608541223483,0.178321019824607,-2.99502561769244));
#7346=CARTESIAN_POINT('Ctrl Pts',(-24.7665915611397,0.222335311776172,-2.99207181620779));
#7347=CARTESIAN_POINT('Ctrl Pts',(-24.7780288192454,0.287837360410405,-2.98624162780084));
#7348=CARTESIAN_POINT('Ctrl Pts',(-24.7823197307722,0.309606561385101,-2.98406194825969));
#7349=CARTESIAN_POINT('Ctrl Pts',(-24.7894679779365,0.34210979841364,-2.98045092915735));
#7350=CARTESIAN_POINT('Ctrl Pts',(-24.7919724393738,0.352930055186471,-2.97918882741414));
#7351=CARTESIAN_POINT('Ctrl Pts',(-24.7972214032702,0.374523340751588,-2.97655141398561));
#7352=CARTESIAN_POINT('Ctrl Pts',(-24.7999681707864,0.38530289681448,-2.97517498996412));
#7353=CARTESIAN_POINT('Ctrl Pts',(-24.8085247289755,0.417396325006842,-2.97090101111402));
#7354=CARTESIAN_POINT('Ctrl Pts',(-24.8146611612218,0.438519664833834,-2.96785340267611));
#7355=CARTESIAN_POINT('Ctrl Pts',(-24.827780795185,0.480245605735748,-2.96138777142348));
#7356=CARTESIAN_POINT('Ctrl Pts',(-24.8347634091537,0.500846985261602,-2.95797002138279));
#7357=CARTESIAN_POINT('Ctrl Pts',(-24.8569585745012,0.56188530630259,-2.94720211826449));
#7358=CARTESIAN_POINT('Ctrl Pts',(-24.8734157851973,0.601558415893423,-2.93933707448591));
#7359=CARTESIAN_POINT('Ctrl Pts',(-24.9005699650057,0.659577946472717,-2.92666307786021));
#7360=CARTESIAN_POINT('Ctrl Pts',(-24.9100343005407,0.678670330222986,-2.92229185258577));
#7361=CARTESIAN_POINT('Ctrl Pts',(-24.9297925040438,0.716356052195618,-2.91328291034591));
#7362=CARTESIAN_POINT('Ctrl Pts',(-24.9400941970776,0.734962854491031,-2.90864166879987));
#7363=CARTESIAN_POINT('Ctrl Pts',(-24.9615143509208,0.771630108002674,-2.8991297911222));
#7364=CARTESIAN_POINT('Ctrl Pts',(-24.9725542617936,0.789558390564705,-2.89429401664935));
#7365=CARTESIAN_POINT('Ctrl Pts',(-24.9953081681755,0.824675412874893,-2.88448450367961));
#7366=CARTESIAN_POINT('Ctrl Pts',(-25.0070176561689,0.841856330313487,-2.87951274183947));
#7367=CARTESIAN_POINT('Ctrl Pts',(-25.0431332882325,0.892293349065714,-2.86444629839691));
#7368=CARTESIAN_POINT('Ctrl Pts',(-25.0685240643679,0.924446248154153,-2.85419987571196));
#7369=CARTESIAN_POINT('Ctrl Pts',(-25.1085917532924,0.970519332950315,-2.83872559859403));
#7370=CARTESIAN_POINT('Ctrl Pts',(-25.1222785365167,0.985516952511361,-2.83355000263622));
#7371=CARTESIAN_POINT('Ctrl Pts',(-25.1503245087481,1.01479156009321,-2.82319808714425));
#7372=CARTESIAN_POINT('Ctrl Pts',(-25.1646905450052,1.02907433729269,-2.81801945772865));
#7373=CARTESIAN_POINT('Ctrl Pts',(-25.1940839460452,1.05688985201169,-2.80770598732435));
#7374=CARTESIAN_POINT('Ctrl Pts',(-25.2091788350748,1.07047868451994,-2.80254912945966));
#7375=CARTESIAN_POINT('Ctrl Pts',(-25.2397857985023,1.09666875082296,-2.79240445901191));
#7376=CARTESIAN_POINT('Ctrl Pts',(-25.255320223101,1.10929658351523,-2.78740768552752));
#7377=CARTESIAN_POINT('Ctrl Pts',(-25.2868469170525,1.13362940492585,-2.77760057560581));
#7378=CARTESIAN_POINT('Ctrl Pts',(-25.302839623016,1.1453353693059,-2.77278994432858));
#7379=CARTESIAN_POINT('Ctrl Pts',(-25.3352860491081,1.16783592991972,-2.76338858760641));
#7380=CARTESIAN_POINT('Ctrl Pts',(-25.3517397751987,1.17863049873126,-2.75879782839759));
#7381=CARTESIAN_POINT('Ctrl Pts',(-25.4018014264425,1.20964993058027,-2.74540766718038));
#7382=CARTESIAN_POINT('Ctrl Pts',(-25.4361157965431,1.22851722530087,-2.7369879943305));
#7383=CARTESIAN_POINT('Ctrl Pts',(-25.4890319606085,1.25402748115623,-2.72534609489846));
#7384=CARTESIAN_POINT('Ctrl Pts',(-25.5069294362475,1.26207118462113,-2.72162720547796));
#7385=CARTESIAN_POINT('Ctrl Pts',(-25.5341341065867,1.2734147976899,-2.71632858891394));
#7386=CARTESIAN_POINT('Ctrl Pts',(-25.5432727036745,1.27707929627405,-2.71460725980808));
#7387=CARTESIAN_POINT('Ctrl Pts',(-25.5616696134459,1.28416319515222,-2.71126336921716));
#7388=CARTESIAN_POINT('Ctrl Pts',(-25.5709426986925,1.28758734347614,-2.70963852456332));
#7389=CARTESIAN_POINT('Ctrl Pts',(-25.5987920948568,1.29743244195315,-2.70494558321287));
#7390=CARTESIAN_POINT('Ctrl Pts',(-25.617433882299,1.30344363716718,-2.70205116137012));
#7391=CARTESIAN_POINT('Ctrl Pts',(-25.6548879621502,1.31438372733535,-2.69674641877481));
#7392=CARTESIAN_POINT('Ctrl Pts',(-25.6736968490448,1.31931173160549,-2.69433651551851));
#7393=CARTESIAN_POINT('Ctrl Pts',(-25.7303690237763,1.33248274213306,-2.68786059982171));
#7394=CARTESIAN_POINT('Ctrl Pts',(-25.7684773832559,1.33911643529057,-2.6845486252675));
#7395=CARTESIAN_POINT('Ctrl Pts',(-25.8261391213393,1.34582410918547,-2.68118864483475));
#7396=CARTESIAN_POINT('Ctrl Pts',(-25.8454430068625,1.34751862690546,-2.68033657178925));
#7397=CARTESIAN_POINT('Ctrl Pts',(-25.8842203794928,1.34980853567156,-2.67918411053142));
#7398=CARTESIAN_POINT('Ctrl Pts',(-25.9037051371427,1.35040321450497,-2.67888411665588));
#7399=CARTESIAN_POINT('Ctrl Pts',(-25.9428031440834,1.35047173299046,-2.67884957398268));
#7400=CARTESIAN_POINT('Ctrl Pts',(-25.9625262788924,1.34993763378489,-2.67911903945912));
#7401=CARTESIAN_POINT('Ctrl Pts',(-26.001675179068,1.34774256849849,-2.68022395142751));
#7402=CARTESIAN_POINT('Ctrl Pts',(-26.0211401464231,1.34608753889996,-2.68105638390197));
#7403=CARTESIAN_POINT('Ctrl Pts',(-26.0598521561959,1.34168374443806,-2.68326288816888));
#7404=CARTESIAN_POINT('Ctrl Pts',(-26.0790999491839,1.33893558390627,-2.68463664029073));
#7405=CARTESIAN_POINT('Ctrl Pts',(-26.1173832731121,1.33236285214625,-2.68790468740719));
#7406=CARTESIAN_POINT('Ctrl Pts',(-26.1364187960914,1.32853823376571,-2.68979898789909));
#7407=CARTESIAN_POINT('Ctrl Pts',(-26.1932112333693,1.31546132541519,-2.69623160867151));
#7408=CARTESIAN_POINT('Ctrl Pts',(-26.230658868257,1.30460568802835,-2.70152164206104));
#7409=CARTESIAN_POINT('Ctrl Pts',(-26.2769394358952,1.28835579481113,-2.70927322407079));
#7410=CARTESIAN_POINT('Ctrl Pts',(-26.2861736873588,1.28496804550344,-2.71088197061785));
#7411=CARTESIAN_POINT('Ctrl Pts',(-26.3045801226384,1.27792632816734,-2.71420859259991));
#7412=CARTESIAN_POINT('Ctrl Pts',(-26.3137696612827,1.2742643583807,-2.71593014837301));
#7413=CARTESIAN_POINT('Ctrl Pts',(-26.3411343470425,1.26292005406289,-2.72123342520569));
#7414=CARTESIAN_POINT('Ctrl Pts',(-26.3591086288947,1.25488236548528,-2.72495256846717));
#7415=CARTESIAN_POINT('Ctrl Pts',(-26.3945730991822,1.23786441433936,-2.73272536195925));
#7416=CARTESIAN_POINT('Ctrl Pts',(-26.4120574252086,1.22888679609907,-2.73677778918298));
#7417=CARTESIAN_POINT('Ctrl Pts',(-26.4465443911629,1.21000870437875,-2.74517655409932));
#7418=CARTESIAN_POINT('Ctrl Pts',(-26.4635470144595,1.20010820517652,-2.74952291627503));
#7419=CARTESIAN_POINT('Ctrl Pts',(-26.4970806133762,1.1793905896332,-2.75847308374743));
#7420=CARTESIAN_POINT('Ctrl Pts',(-26.5136115807888,1.16857346524795,-2.76307691198199));
#7421=CARTESIAN_POINT('Ctrl Pts',(-26.546208083381,1.14602103189425,-2.77250675337683));
#7422=CARTESIAN_POINT('Ctrl Pts',(-26.5622736983626,1.1342856634169,-2.77733281570969));
#7423=CARTESIAN_POINT('Ctrl Pts',(-26.5939416429695,1.10988763337468,-2.7871725670388));
#7424=CARTESIAN_POINT('Ctrl Pts',(-26.609547564207,1.09722193187052,-2.79218745199254));
#7425=CARTESIAN_POINT('Ctrl Pts',(-26.6402813438902,1.0709572172429,-2.8023664037371));
#7426=CARTESIAN_POINT('Ctrl Pts',(-26.655295080658,1.05745634546246,-2.80749236059604));
#7427=CARTESIAN_POINT('Ctrl Pts',(-26.6846548548111,1.02971401041124,-2.81778570291711));
#7428=CARTESIAN_POINT('Ctrl Pts',(-26.698997953854,1.01547501212972,-2.82295214467571));
#7429=CARTESIAN_POINT('Ctrl Pts',(-26.7270253212179,0.986266221033504,-2.83328911051858));
#7430=CARTESIAN_POINT('Ctrl Pts',(-26.7407095447861,0.971296396677911,-2.83845969056953));
#7431=CARTESIAN_POINT('Ctrl Pts',(-26.7807872610901,0.925288863725479,-2.85392633511737));
#7432=CARTESIAN_POINT('Ctrl Pts',(-26.8062107356642,0.893151941339911,-2.864178670324));
#7433=CARTESIAN_POINT('Ctrl Pts',(-26.8423947744529,0.84270457925161,-2.87926472137709));
#7434=CARTESIAN_POINT('Ctrl Pts',(-26.8541358893937,0.825504953419084,-2.88424727122285));
#7435=CARTESIAN_POINT('Ctrl Pts',(-26.8712465648999,0.799139107619223,-2.89162033090013));
#7436=CARTESIAN_POINT('Ctrl Pts',(-26.8768710845513,0.79024832752982,-2.89406322620423));
#7437=CARTESIAN_POINT('Ctrl Pts',(-26.8879472162261,0.772282090199624,-2.89890928529195));
#7438=CARTESIAN_POINT('Ctrl Pts',(-26.8934095805383,0.763187949365322,-2.9013172405501));
#7439=CARTESIAN_POINT('Ctrl Pts',(-26.9094752397211,0.735724969537463,-2.90844874441802));
#7440=CARTESIAN_POINT('Ctrl Pts',(-26.9197553059395,0.717185246436085,-2.91307852354811));
#7441=CARTESIAN_POINT('Ctrl Pts',(-26.939491662068,0.679606241243716,-2.92207399934037));
#7442=CARTESIAN_POINT('Ctrl Pts',(-26.9489441843561,0.660573675186059,-2.92643805302077));
#7443=CARTESIAN_POINT('Ctrl Pts',(-26.9760664924628,0.602745972669876,-2.93909208245403));
#7444=CARTESIAN_POINT('Ctrl Pts',(-26.9925039932974,0.563222492320482,-2.94694446393472));
#7445=CARTESIAN_POINT('Ctrl Pts',(-27.0220719282814,0.482184935663522,-2.96128319208414));
#7446=CARTESIAN_POINT('Ctrl Pts',(-27.0352038812473,0.440658278132658,-2.96777086803717));
#7447=CARTESIAN_POINT('Ctrl Pts',(-27.0523220500515,0.376834051179658,-2.97631783456127));
#7448=CARTESIAN_POINT('Ctrl Pts',(-27.0576008937577,0.355274612711088,-2.97897112077082));
#7449=CARTESIAN_POINT('Ctrl Pts',(-27.0672604256937,0.311662928430509,-2.98384906046174));
#7450=CARTESIAN_POINT('Ctrl Pts',(-27.0716118507556,0.28974195783202,-2.98605887165636));
#7451=CARTESIAN_POINT('Ctrl Pts',(-27.0793664061891,0.245626216202852,-2.99001098961276));
#7452=CARTESIAN_POINT('Ctrl Pts',(-27.0827665013565,0.223449220869779,-2.99175175446374));
#7453=CARTESIAN_POINT('Ctrl Pts',(-27.0886129441394,0.178789236716058,-2.99475258363014));
#7454=CARTESIAN_POINT('Ctrl Pts',(-27.0910452438611,0.156404759559941,-2.99600543335325));
#7455=CARTESIAN_POINT('Ctrl Pts',(-27.0968540554839,0.0893800728363459,
-2.99900191231137));
#7456=CARTESIAN_POINT('Ctrl Pts',(-27.0987766251388,0.044721791781682,-2.99999958185766));
#7457=CARTESIAN_POINT('Ctrl Pts',(-27.0987813865579,-0.0221932547862428,
-3.00000207062791));
#7458=CARTESIAN_POINT('Ctrl Pts',(-27.098302980501,-0.0444882044529787,
-2.99975417679133));
#7459=CARTESIAN_POINT('Ctrl Pts',(-27.0963851499708,-0.0890579606384743,
-2.99876191230976));
#7460=CARTESIAN_POINT('Ctrl Pts',(-27.0949457527391,-0.111332767632209,
-2.99801754221172));
#7461=CARTESIAN_POINT('Ctrl Pts',(-27.091097912228,-0.155862099946069,-2.99603257401337));
#7462=CARTESIAN_POINT('Ctrl Pts',(-27.0886882785475,-0.178121325914285,
-2.99479136150237));
#7463=CARTESIAN_POINT('Ctrl Pts',(-27.0828893311938,-0.222600421497835,
-2.99181469259339));
#7464=CARTESIAN_POINT('Ctrl Pts',(-27.0794844211542,-0.244888534479487,
-2.99007132802239));
#7465=CARTESIAN_POINT('Ctrl Pts',(-27.0717763207677,-0.288870061738491,
-2.98614250919086));
#7466=CARTESIAN_POINT('Ctrl Pts',(-27.0674611935747,-0.310670506014757,
-2.98395091125391));
#7467=CARTESIAN_POINT('Ctrl Pts',(-27.0579367437935,-0.353839565051261,
-2.9791402804281));
#7468=CARTESIAN_POINT('Ctrl Pts',(-27.0527261874502,-0.37521860103612,-2.97652060572815));
#7469=CARTESIAN_POINT('Ctrl Pts',(-27.0357699204893,-0.438751951157215,
-2.96805162738344));
#7470=CARTESIAN_POINT('Ctrl Pts',(-27.022699391642,-0.480310643319726,-2.96159083395379));
#7471=CARTESIAN_POINT('Ctrl Pts',(-27.0004758229384,-0.541446694763503,
-2.95080875849622));
#7472=CARTESIAN_POINT('Ctrl Pts',(-26.992623681753,-0.561640072316635,-2.94702942050088));
#7473=CARTESIAN_POINT('Ctrl Pts',(-26.9801909795193,-0.591614335345471,
-2.94110596088858));
#7474=CARTESIAN_POINT('Ctrl Pts',(-26.9759332605878,-0.601562265182988,
-2.9390870305072));
#7475=CARTESIAN_POINT('Ctrl Pts',(-26.9671990237161,-0.621350626541995,
-2.93496737112459));
#7476=CARTESIAN_POINT('Ctrl Pts',(-26.9627163520765,-0.631203409825244,
-2.93286380405279));
#7477=CARTESIAN_POINT('Ctrl Pts',(-26.9490003388169,-0.660466615132212,
-2.92646369421333));
#7478=CARTESIAN_POINT('Ctrl Pts',(-26.9394866261483,-0.679617007741934,
-2.92207164107701));
#7479=CARTESIAN_POINT('Ctrl Pts',(-26.9197263731453,-0.717239156030648,
-2.91306539958487));
#7480=CARTESIAN_POINT('Ctrl Pts',(-26.9094813066202,-0.735708225799579,
-2.9084518514383));
#7481=CARTESIAN_POINT('Ctrl Pts',(-26.8776651907974,-0.790114397662374,
-2.8943275255928));
#7482=CARTESIAN_POINT('Ctrl Pts',(-26.855015951808,-0.825052668578734,-2.88453262436396));
#7483=CARTESIAN_POINT('Ctrl Pts',(-26.8188828130475,-0.875511458559026,
-2.86945918682943));
#7484=CARTESIAN_POINT('Ctrl Pts',(-26.806477865951,-0.892005672721584,-2.86437109863275));
#7485=CARTESIAN_POINT('Ctrl Pts',(-26.7809370903558,-0.924343794681306,
-2.85409960048902));
#7486=CARTESIAN_POINT('Ctrl Pts',(-26.7678062754663,-0.940181784684746,
-2.84891809889913));
#7487=CARTESIAN_POINT('Ctrl Pts',(-26.747534952965,-0.963465362975884,-2.8410930742898));
#7488=CARTESIAN_POINT('Ctrl Pts',(-26.7406847515848,-0.971143336910778,
-2.8384772090519));
#7489=CARTESIAN_POINT('Ctrl Pts',(-26.726866828362,-0.986257778221383,-2.8332609577602));
#7490=CARTESIAN_POINT('Ctrl Pts',(-26.7198864405152,-0.993708965489595,
-2.83065565931378));
#7491=CARTESIAN_POINT('Ctrl Pts',(-26.6987545667654,-1.01572267126074,-2.82286342050641));
#7492=CARTESIAN_POINT('Ctrl Pts',(-26.6843929425923,-1.02996804274084,-2.81769254606288));
#7493=CARTESIAN_POINT('Ctrl Pts',(-26.6405196961263,-1.07140451601385,-2.80231490014363));
#7494=CARTESIAN_POINT('Ctrl Pts',(-26.6101990167324,-1.09732522138671,-2.79223355729095));
#7495=CARTESIAN_POINT('Ctrl Pts',(-26.5630920876351,-1.13367314163992,-2.77758248050925));
#7496=CARTESIAN_POINT('Ctrl Pts',(-26.5471176954077,-1.14536678978724,-2.77277705423988));
#7497=CARTESIAN_POINT('Ctrl Pts',(-26.5146128603087,-1.1679042027731,-2.76335982199195));
#7498=CARTESIAN_POINT('Ctrl Pts',(-26.4980824626504,-1.17874802188457,-2.75874796251914));
#7499=CARTESIAN_POINT('Ctrl Pts',(-26.4644489769846,-1.19957326674857,-2.74975657993441));
#7500=CARTESIAN_POINT('Ctrl Pts',(-26.4473526605441,-1.20955077156384,-2.74537877233406));
#7501=CARTESIAN_POINT('Ctrl Pts',(-26.4212418428209,-1.22386659438306,-2.73901196687351));
#7502=CARTESIAN_POINT('Ctrl Pts',(-26.4124621517901,-1.22852809048201,-2.73692383614116));
#7503=CARTESIAN_POINT('Ctrl Pts',(-26.3948579023758,-1.23757356026447,-2.73284557774275));
#7504=CARTESIAN_POINT('Ctrl Pts',(-26.3860148872853,-1.24196849424177,-2.73085066873683));
#7505=CARTESIAN_POINT('Ctrl Pts',(-26.341645261955,-1.26327266721301,-2.72112112107027));
#7506=CARTESIAN_POINT('Ctrl Pts',(-26.3055755853367,-1.27824593843012,-2.71409299783002));
#7507=CARTESIAN_POINT('Ctrl Pts',(-26.2323061069552,-1.30408058177654,-2.70177489330742));
#7508=CARTESIAN_POINT('Ctrl Pts',(-26.1951017095151,-1.314947120491,-2.69648267860914));
#7509=CARTESIAN_POINT('Ctrl Pts',(-26.1384101250037,-1.32811617463851,-2.69000746444321));
#7510=CARTESIAN_POINT('Ctrl Pts',(-26.1193652332726,-1.33198320784822,-2.68809291154563));
#7511=CARTESIAN_POINT('Ctrl Pts',(-26.0809718851876,-1.33864980310861,-2.68477922262698));
#7512=CARTESIAN_POINT('Ctrl Pts',(-26.0616267484912,-1.34144867007466,-2.68338047067986));
#7513=CARTESIAN_POINT('Ctrl Pts',(-26.032363761062,-1.344825402147,-2.68168886075705));
#7514=CARTESIAN_POINT('Ctrl Pts',(-26.0225572765905,-1.34581398544559,-2.6811927471385));
#7515=CARTESIAN_POINT('Ctrl Pts',(-26.0029866880182,-1.3475022070275,-2.68034468497322));
#7516=CARTESIAN_POINT('Ctrl Pts',(-25.9932072525691,-1.34820413161833,-2.67999159504196));
#7517=CARTESIAN_POINT('Ctrl Pts',(-25.9639248763077,-1.34988314454028,-2.6791465090366));
#7518=CARTESIAN_POINT('Ctrl Pts',(-25.944430256616,-1.35043954651562,-2.67886577671176));
#7519=CARTESIAN_POINT('Ctrl Pts',(-25.8861245439706,-1.35043780955491,-2.67886672345498));
#7520=CARTESIAN_POINT('Ctrl Pts',(-25.8474103812661,-1.34822168461924,-2.67998726078285));
#7521=CARTESIAN_POINT('Ctrl Pts',(-25.7896108997839,-1.34161043104657,-2.68329952853648));
#7522=CARTESIAN_POINT('Ctrl Pts',(-25.77038745646,-1.33885814096474,-2.68467529043326));
#7523=CARTESIAN_POINT('Ctrl Pts',(-25.7320267290187,-1.33225068682403,-2.68796030874541));
#7524=CARTESIAN_POINT('Ctrl Pts',(-25.7128830247106,-1.32839365293775,-2.68987049972103));
#7525=CARTESIAN_POINT('Ctrl Pts',(-25.684251748041,-1.3217762322719,-2.69312505274073));
#7526=CARTESIAN_POINT('Ctrl Pts',(-25.6747141290368,-1.31942923189442,-2.69427597594583));
#7527=CARTESIAN_POINT('Ctrl Pts',(-25.6556602502347,-1.31445363734785,-2.69670691417442));
#7528=CARTESIAN_POINT('Ctrl Pts',(-25.6461499439872,-1.31182592199725,-2.69798646989668));
#7529=CARTESIAN_POINT('Ctrl Pts',(-25.6178199688841,-1.30356690507149,-2.70199177974631));
#7530=CARTESIAN_POINT('Ctrl Pts',(-25.5991462839436,-1.29754850153217,-2.70488980770929));
#7531=CARTESIAN_POINT('Ctrl Pts',(-25.5622141869212,-1.28451064624858,-2.71110556040654));
#7532=CARTESIAN_POINT('Ctrl Pts',(-25.5439551422566,-1.27749140423904,-2.7144231880909));
#7533=CARTESIAN_POINT('Ctrl Pts',(-25.5078398888184,-1.26246846951839,-2.72144279020549));
#7534=CARTESIAN_POINT('Ctrl Pts',(-25.4899837037464,-1.25446472257529,-2.72514479532609));
#7535=CARTESIAN_POINT('Ctrl Pts',(-25.4370072942282,-1.22898847560419,-2.7367763145851));
#7536=CARTESIAN_POINT('Ctrl Pts',(-25.4024760017175,-1.21005101589909,-2.74523245622064));
#7537=CARTESIAN_POINT('Ctrl Pts',(-25.3602838735484,-1.18392877826527,-2.75651122868635));
#7538=CARTESIAN_POINT('Ctrl Pts',(-25.3518919706823,-1.1785784585637,-2.75880349026456));
#7539=CARTESIAN_POINT('Ctrl Pts',(-25.3352100824015,-1.16763411776592,-2.76345337348231));
#7540=CARTESIAN_POINT('Ctrl Pts',(-25.3269100051743,-1.16203215951807,-2.76581417940247));
#7541=CARTESIAN_POINT('Ctrl Pts',(-25.3022695725318,-1.1449302461251,-2.77295794310451));
#7542=CARTESIAN_POINT('Ctrl Pts',(-25.2861657292169,-1.1331226072542,-2.77780759607732));
#7543=CARTESIAN_POINT('Ctrl Pts',(-25.2545675218788,-1.10869580205534,-2.78764693628012));
#7544=CARTESIAN_POINT('Ctrl Pts',(-25.2390758775543,-1.09607878865392,-2.7926357760188));
#7545=CARTESIAN_POINT('Ctrl Pts',(-25.208692728647,-1.07004449005285,-2.80271440082356));
#7546=CARTESIAN_POINT('Ctrl Pts',(-25.193801243974,-1.05662718870003,-2.80780421768085));
#7547=CARTESIAN_POINT('Ctrl Pts',(-25.1646090505302,-1.02899230331322,-2.81804902565378));
#7548=CARTESIAN_POINT('Ctrl Pts',(-25.150308350114,-1.0147747185966,-2.82320404678685));
#7549=CARTESIAN_POINT('Ctrl Pts',(-25.1222934624824,-0.985532507337774,
-2.83354449797841));
#7550=CARTESIAN_POINT('Ctrl Pts',(-25.1085792726074,-0.970507895413089,
-2.83872995787953));
#7551=CARTESIAN_POINT('Ctrl Pts',(-25.0817381947277,-0.939637998238792,
-2.84909699750195));
#7552=CARTESIAN_POINT('Ctrl Pts',(-25.0686119208846,-0.923793044275975,
-2.85427840682449));
#7553=CARTESIAN_POINT('Ctrl Pts',(-25.0493655924709,-0.899393527288515,
-2.86202245059147));
#7554=CARTESIAN_POINT('Ctrl Pts',(-25.0430172047533,-0.891144919357547,
-2.86460202126226));
#7555=CARTESIAN_POINT('Ctrl Pts',(-25.0305204210295,-0.874501923571611,
-2.86972650110557));
#7556=CARTESIAN_POINT('Ctrl Pts',(-25.02437110194,-0.866107944767961,-2.87227157889308));
#7557=CARTESIAN_POINT('Ctrl Pts',(-24.9941173036171,-0.823768140450459,
-2.88490209785398));
#7558=CARTESIAN_POINT('Ctrl Pts',(-24.971471952131,-0.788729223015765,-2.89470441040781));
#7559=CARTESIAN_POINT('Ctrl Pts',(-24.9292309034491,-0.716312201964237,
-2.91346931208067));
#7560=CARTESIAN_POINT('Ctrl Pts',(-24.9096333854723,-0.678934856512817,
-2.92243312349527));
#7561=CARTESIAN_POINT('Ctrl Pts',(-24.882541170584,-0.621060652496466,-2.93507771188247));
#7562=CARTESIAN_POINT('Ctrl Pts',(-24.8738951241541,-0.601467423657379,
-2.93915911726366));
#7563=CARTESIAN_POINT('Ctrl Pts',(-24.8573856909762,-0.561660850722057,
-2.94702500788258));
#7564=CARTESIAN_POINT('Ctrl Pts',(-24.8495218895994,-0.541445422596667,
-2.95080973422482));
#7565=CARTESIAN_POINT('Ctrl Pts',(-24.8383292807319,-0.510647491444323,
-2.95624018705409));
#7566=CARTESIAN_POINT('Ctrl Pts',(-24.8346940039926,-0.500285853504755,
-2.95801168194031));
#7567=CARTESIAN_POINT('Ctrl Pts',(-24.8276504459147,-0.479468083601724,
-2.96145728412087));
#7568=CARTESIAN_POINT('Ctrl Pts',(-24.8242483365591,-0.469031804392169,
-2.96312833452968));
#7569=CARTESIAN_POINT('Ctrl Pts',(-24.8143971656437,-0.437635791555516,
-2.96798415471264));
#7570=CARTESIAN_POINT('Ctrl Pts',(-24.8082915227193,-0.416559647886908,
-2.97101715178475));
#7571=CARTESIAN_POINT('Ctrl Pts',(-24.7970093173975,-0.374165786036183,
-2.97665328568467));
#7572=CARTESIAN_POINT('Ctrl Pts',(-24.7918298385069,-0.352840123671072,
-2.97925785882102));
#7573=CARTESIAN_POINT('Ctrl Pts',(-24.782389163039,-0.309931323851523,-2.98402682340998));
#7574=CARTESIAN_POINT('Ctrl Pts',(-24.7781279721287,-0.288348186260508,
-2.98619122824603));
#7575=CARTESIAN_POINT('Ctrl Pts',(-24.7705258708633,-0.244922725747239,
-2.99006614582328));
#7576=CARTESIAN_POINT('Ctrl Pts',(-24.7671849516661,-0.223080406167035,
-2.99177667236476));
#7577=CARTESIAN_POINT('Ctrl Pts',(-24.7614323434624,-0.17913315210593,-2.99472933868235));
#7578=CARTESIAN_POINT('Ctrl Pts',(-24.7590206303916,-0.157028224677867,
-2.99597149337493));
#7579=CARTESIAN_POINT('Ctrl Pts',(-24.7551426261223,-0.11255051417061,-2.99797188287434));
#7580=CARTESIAN_POINT('Ctrl Pts',(-24.7536766612853,-0.0901766051585172,
-2.99872994324477));
#7581=CARTESIAN_POINT('Ctrl Pts',(-24.7522036848644,-0.0564128512141614,
-2.99949202836052));
#7582=CARTESIAN_POINT('Ctrl Pts',(-24.7518340087419,-0.0451069176116392,
-2.9996834086165));
#7583=CARTESIAN_POINT('Ctrl Pts',(-24.751342340005,-0.0225174807117986,
-2.99993797771742));
#7584=CARTESIAN_POINT('Ctrl Pts',(-24.751219987252,-0.0112452307973086,
-3.00000135224878));
#7585=CARTESIAN_POINT('Ctrl Pts',(-24.7512201965622,1.27647978108407E-15,
-3.00000124311957));
#7586=CARTESIAN_POINT('Ctrl Pts',(-24.9250015605239,9.19874578470569E-16,
-2.60754908509523));
#7587=CARTESIAN_POINT('Ctrl Pts',(-24.9250019171665,0.0166541334801639,
-2.60754889538879));
#7588=CARTESIAN_POINT('Ctrl Pts',(-24.9254176382407,0.0332580512905832,
-2.60732913473254));
#7589=CARTESIAN_POINT('Ctrl Pts',(-24.9270664927659,0.0663302887433929,
-2.60645878753387));
#7590=CARTESIAN_POINT('Ctrl Pts',(-24.9282993169708,0.0828048613803127,
-2.60580837511734));
#7591=CARTESIAN_POINT('Ctrl Pts',(-24.9332091568075,0.13204629231987,-2.60322435771041));
#7592=CARTESIAN_POINT('Ctrl Pts',(-24.9380971518304,0.164638771132329,-2.60065696465499));
#7593=CARTESIAN_POINT('Ctrl Pts',(-24.9478410920693,0.213142882820904,-2.59558946593898));
#7594=CARTESIAN_POINT('Ctrl Pts',(-24.9514967222119,0.229262924518064,-2.59369492625984));
#7595=CARTESIAN_POINT('Ctrl Pts',(-24.957586651506,0.253331494462504,-2.59055629104136));
#7596=CARTESIAN_POINT('Ctrl Pts',(-24.9597203204629,0.261343868943604,-2.58945929408072));
#7597=CARTESIAN_POINT('Ctrl Pts',(-24.9641921606581,0.277333645699331,-2.58716690003976));
#7598=CARTESIAN_POINT('Ctrl Pts',(-24.9665322616052,0.28531588140159,-2.58597053613621));
#7599=CARTESIAN_POINT('Ctrl Pts',(-24.9738219975603,0.309080988873586,-2.58225566779539));
#7600=CARTESIAN_POINT('Ctrl Pts',(-24.9790499139481,0.32472277192427,-2.57960673936175));
#7601=CARTESIAN_POINT('Ctrl Pts',(-24.9902271496198,0.355620732215228,-2.57398692473799));
#7602=CARTESIAN_POINT('Ctrl Pts',(-24.9961759681728,0.37087600490021,-2.57101627563854));
#7603=CARTESIAN_POINT('Ctrl Pts',(-25.015085077571,0.416074736889802,-2.5616570008748));
#7604=CARTESIAN_POINT('Ctrl Pts',(-25.0291057524579,0.445452580460475,-2.55482084113839));
#7605=CARTESIAN_POINT('Ctrl Pts',(-25.0522396804357,0.48841590527102,-2.54380482293415));
#7606=CARTESIAN_POINT('Ctrl Pts',(-25.060302794776,0.502553770162824,-2.54000542968693));
#7607=CARTESIAN_POINT('Ctrl Pts',(-25.0771357413066,0.530459957917388,-2.53217501323324));
#7608=CARTESIAN_POINT('Ctrl Pts',(-25.0859122400396,0.544238250893843,-2.5281409265225));
#7609=CARTESIAN_POINT('Ctrl Pts',(-25.1041610805409,0.571390265168163,-2.51987336730303));
#7610=CARTESIAN_POINT('Ctrl Pts',(-25.113566501909,0.5846661158911,-2.51567019594392));
#7611=CARTESIAN_POINT('Ctrl Pts',(-25.1329516291768,0.610670187636857,-2.50714393728714));
#7612=CARTESIAN_POINT('Ctrl Pts',(-25.1429274949106,0.62339261625794,-2.50282256806535));
#7613=CARTESIAN_POINT('Ctrl Pts',(-25.1736961072169,0.660741109040548,-2.48972707655348));
#7614=CARTESIAN_POINT('Ctrl Pts',(-25.195327708338,0.684550254569154,-2.48082106354485));
#7615=CARTESIAN_POINT('Ctrl Pts',(-25.2294632644966,0.718667264605287,-2.46737109007097));
#7616=CARTESIAN_POINT('Ctrl Pts',(-25.2411236814041,0.729772966325552,-2.46287255176687));
#7617=CARTESIAN_POINT('Ctrl Pts',(-25.2650173694561,0.75145074381943,-2.45387484623858));
#7618=CARTESIAN_POINT('Ctrl Pts',(-25.2772564740961,0.762027106466311,-2.44937367130548));
#7619=CARTESIAN_POINT('Ctrl Pts',(-25.3022981003744,0.782624429155002,-2.44040938158116));
#7620=CARTESIAN_POINT('Ctrl Pts',(-25.3151581491073,0.792686927403694,-2.43592713010271));
#7621=CARTESIAN_POINT('Ctrl Pts',(-25.3412336664868,0.812080609394974,-2.42710955837505));
#7622=CARTESIAN_POINT('Ctrl Pts',(-25.3544681763255,0.821431489558632,-2.42276644946543));
#7623=CARTESIAN_POINT('Ctrl Pts',(-25.3813272555676,0.839449886111474,-2.41424227949637));
#7624=CARTESIAN_POINT('Ctrl Pts',(-25.3949521969405,0.848118124975925,-2.41006096216709));
#7625=CARTESIAN_POINT('Ctrl Pts',(-25.4225948394221,0.864779736753664,-2.40188946584664));
#7626=CARTESIAN_POINT('Ctrl Pts',(-25.4366125456109,0.872773089361185,-2.39789925750829));
#7627=CARTESIAN_POINT('Ctrl Pts',(-25.4792624301743,0.895742905086413,-2.38626076145437));
#7628=CARTESIAN_POINT('Ctrl Pts',(-25.5084964623614,0.909714092086876,-2.37894252774089));
#7629=CARTESIAN_POINT('Ctrl Pts',(-25.5535782411859,0.928604376053527,-2.36882359052986));
#7630=CARTESIAN_POINT('Ctrl Pts',(-25.5688259457879,0.934560719395066,-2.36559119630037));
#7631=CARTESIAN_POINT('Ctrl Pts',(-25.5920028890314,0.942960637972606,-2.36098573061775));
#7632=CARTESIAN_POINT('Ctrl Pts',(-25.599788491408,0.945674190484414,-2.35948958119257));
#7633=CARTESIAN_POINT('Ctrl Pts',(-25.6154616875292,0.950919800805258,-2.35658312944662));
#7634=CARTESIAN_POINT('Ctrl Pts',(-25.6233618667185,0.953455374519274,-2.35517084263495));
#7635=CARTESIAN_POINT('Ctrl Pts',(-25.6470880823365,0.960745646595264,-2.35109181935035));
#7636=CARTESIAN_POINT('Ctrl Pts',(-25.6629699013087,0.965196922396597,-2.3485760380501));
#7637=CARTESIAN_POINT('Ctrl Pts',(-25.694878800485,0.973298033223304,-2.34396524772702));
#7638=CARTESIAN_POINT('Ctrl Pts',(-25.7109029793721,0.976947208699529,-2.34187060158446));
#7639=CARTESIAN_POINT('Ctrl Pts',(-25.7591846810364,0.986700310761385,-2.33624184790048));
#7640=CARTESIAN_POINT('Ctrl Pts',(-25.7916509919276,0.991612544814411,-2.33336313702002));
#7641=CARTESIAN_POINT('Ctrl Pts',(-25.8407757493374,0.996579561426926,-2.33044270026262));
#7642=CARTESIAN_POINT('Ctrl Pts',(-25.8572216409297,0.997834347780408,-2.32970209313936));
#7643=CARTESIAN_POINT('Ctrl Pts',(-25.8902579157094,0.99953001979152,-2.32870039378829));
#7644=CARTESIAN_POINT('Ctrl Pts',(-25.9068579008084,0.999970378057446,-2.32843964431104));
#7645=CARTESIAN_POINT('Ctrl Pts',(-25.940167339092,1.00002111583352,-2.3284096204183));
#7646=CARTESIAN_POINT('Ctrl Pts',(-25.9569704089505,0.999625616638201,-2.32864383514006));
#7647=CARTESIAN_POINT('Ctrl Pts',(-25.9903232055858,0.998000175999137,-2.32960420547288));
#7648=CARTESIAN_POINT('Ctrl Pts',(-26.0069063303974,0.996774630505938,-2.33032774135208));
#7649=CARTESIAN_POINT('Ctrl Pts',(-26.0398869194724,0.993513631149881,-2.33224559661821));
#7650=CARTESIAN_POINT('Ctrl Pts',(-26.056285023184,0.991478624792932,-2.33343963815292));
#7651=CARTESIAN_POINT('Ctrl Pts',(-26.0889003945458,0.98661153251092,-2.33628016806539));
#7652=CARTESIAN_POINT('Ctrl Pts',(-26.105117655415,0.98377941166941,-2.33792666122146));
#7653=CARTESIAN_POINT('Ctrl Pts',(-26.1535018144213,0.97409599204652,-2.34351778370754));
#7654=CARTESIAN_POINT('Ctrl Pts',(-26.1854052228443,0.96605741829964,-2.34811578904635));
#7655=CARTESIAN_POINT('Ctrl Pts',(-26.2248338237297,0.954024410911557,-2.35485332977763));
#7656=CARTESIAN_POINT('Ctrl Pts',(-26.2327009185887,0.951515790581765,-2.35625162439446));
#7657=CARTESIAN_POINT('Ctrl Pts',(-26.2483822299402,0.946301415592771,-2.35914306656481));
#7658=CARTESIAN_POINT('Ctrl Pts',(-26.2562112318338,0.943589735649575,-2.36063941300517));
#7659=CARTESIAN_POINT('Ctrl Pts',(-26.2795244997708,0.935189305203656,-2.36524892931282));
#7660=CARTESIAN_POINT('Ctrl Pts',(-26.2948376392117,0.929237415872069,-2.36848154417624));
#7661=CARTESIAN_POINT('Ctrl Pts',(-26.325051496053,0.916635663404135,-2.37523752156304));
#7662=CARTESIAN_POINT('Ctrl Pts',(-26.3399472189906,0.909987758386285,-2.37875982107005));
#7663=CARTESIAN_POINT('Ctrl Pts',(-26.3693282937335,0.896008576234029,-2.38605988196961));
#7664=CARTESIAN_POINT('Ctrl Pts',(-26.3838136313699,0.888677280052345,-2.38983766464246));
#7665=CARTESIAN_POINT('Ctrl Pts',(-26.4123824877164,0.873335934871323,-2.39761699508693));
#7666=CARTESIAN_POINT('Ctrl Pts',(-26.426465999434,0.865325879915263,-2.40161856279579));
#7667=CARTESIAN_POINT('Ctrl Pts',(-26.4542364991726,0.848625856496655,-2.40981481750004));
#7668=CARTESIAN_POINT('Ctrl Pts',(-26.4679235551807,0.839935843967827,-2.4140095472354));
#7669=CARTESIAN_POINT('Ctrl Pts',(-26.4949029725259,0.821869160578012,-2.42256208855009));
#7670=CARTESIAN_POINT('Ctrl Pts',(-26.508198393727,0.812490238648992,-2.42692093963487));
#7671=CARTESIAN_POINT('Ctrl Pts',(-26.5343819518632,0.793041279750162,-2.43576830807168));
#7672=CARTESIAN_POINT('Ctrl Pts',(-26.5471728631521,0.783043916212135,-2.44022370093141));
#7673=CARTESIAN_POINT('Ctrl Pts',(-26.5721858410978,0.7625007828935,-2.44917049567471));
#7674=CARTESIAN_POINT('Ctrl Pts',(-26.5844054044419,0.751956838431777,-2.45366107730755));
#7675=CARTESIAN_POINT('Ctrl Pts',(-26.6082832421287,0.7303277978894,-2.46264578885995));
#7676=CARTESIAN_POINT('Ctrl Pts',(-26.6199414783443,0.719242678452873,-2.46713996742475));
#7677=CARTESIAN_POINT('Ctrl Pts',(-26.654085577301,0.685174209401599,-2.48058330680097));
#7678=CARTESIAN_POINT('Ctrl Pts',(-26.6757450357663,0.661376894583318,-2.48949445887106));
#7679=CARTESIAN_POINT('Ctrl Pts',(-26.7065719269914,0.624020742585242,-2.50260699297805));
#7680=CARTESIAN_POINT('Ctrl Pts',(-26.7165747372154,0.611284460442826,-2.50693773894738));
#7681=CARTESIAN_POINT('Ctrl Pts',(-26.7311521296313,0.591760614150662,-2.51334627463049));
#7682=CARTESIAN_POINT('Ctrl Pts',(-26.7359439235075,0.585177012577667,-2.51546959688903));
#7683=CARTESIAN_POINT('Ctrl Pts',(-26.7453802030872,0.571873056438928,-2.51968170745715));
#7684=CARTESIAN_POINT('Ctrl Pts',(-26.7500338491731,0.565138866716572,-2.52177466043333));
#7685=CARTESIAN_POINT('Ctrl Pts',(-26.7637209428383,0.544802595278455,-2.52797323999353));
#7686=CARTESIAN_POINT('Ctrl Pts',(-26.7724790166661,0.531073974286136,-2.53199736377098));
#7687=CARTESIAN_POINT('Ctrl Pts',(-26.7892933503868,0.503246810054306,-2.53981607542183));
#7688=CARTESIAN_POINT('Ctrl Pts',(-26.7973464004641,0.48915324002206,-2.54360923524379));
#7689=CARTESIAN_POINT('Ctrl Pts',(-26.8204531754343,0.446331963437203,-2.55460789831046));
#7690=CARTESIAN_POINT('Ctrl Pts',(-26.8344570585593,0.417064919965781,-2.56143305219686));
#7691=CARTESIAN_POINT('Ctrl Pts',(-26.8596473785478,0.357056801425753,-2.57389602618922));
#7692=CARTESIAN_POINT('Ctrl Pts',(-26.8708351093533,0.326306410018255,-2.57953500168131));
#7693=CARTESIAN_POINT('Ctrl Pts',(-26.8854188856717,0.279044721282978,-2.58696387685386));
#7694=CARTESIAN_POINT('Ctrl Pts',(-26.889916181885,0.263080008230864,-2.58927006723959));
#7695=CARTESIAN_POINT('Ctrl Pts',(-26.8981455932565,0.230785659439779,-2.59350988787546));
#7696=CARTESIAN_POINT('Ctrl Pts',(-26.9018527777375,0.21455323269401,-2.59543061746581));
#7697=CARTESIAN_POINT('Ctrl Pts',(-26.9084592496751,0.181885630631588,-2.5988657298962));
#7698=CARTESIAN_POINT('Ctrl Pts',(-26.9113559512979,0.165463618176976,-2.60037877253407));
#7699=CARTESIAN_POINT('Ctrl Pts',(-26.9163368119689,0.13239300581574,-2.60298704123574));
#7700=CARTESIAN_POINT('Ctrl Pts',(-26.9184090029522,0.115817353571132,-2.60407599650051));
#7701=CARTESIAN_POINT('Ctrl Pts',(-26.9233578038635,0.0661857319676014,
-2.60668048407778));
#7702=CARTESIAN_POINT('Ctrl Pts',(-26.9249957317331,0.0331163807650845,
-2.60754764115517));
#7703=CARTESIAN_POINT('Ctrl Pts',(-26.9249997882108,-0.0164340525421252,
-2.60754980435114));
#7704=CARTESIAN_POINT('Ctrl Pts',(-26.924592211501,-0.0329434099001476,
-2.60733433932483));
#7705=CARTESIAN_POINT('Ctrl Pts',(-26.922958321114,-0.0659472086648998,
-2.60647188023517));
#7706=CARTESIAN_POINT('Ctrl Pts',(-26.9217320306451,-0.0824416504222753,
-2.60582488664724));
#7707=CARTESIAN_POINT('Ctrl Pts',(-26.9184538736218,-0.115415515405943,
-2.6040995866923));
#7708=CARTESIAN_POINT('Ctrl Pts',(-26.9164009929087,-0.13189841944903,-2.60302074629033));
#7709=CARTESIAN_POINT('Ctrl Pts',(-26.911460595836,-0.164835084256706,-2.60043347726539));
#7710=CARTESIAN_POINT('Ctrl Pts',(-26.9085597921968,-0.181339379062668,
-2.59891817499629));
#7711=CARTESIAN_POINT('Ctrl Pts',(-26.9019928975065,-0.213907595706399,
-2.59550331376099));
#7712=CARTESIAN_POINT('Ctrl Pts',(-26.8983166368945,-0.230050772994295,
-2.59359841481876));
#7713=CARTESIAN_POINT('Ctrl Pts',(-26.8902023083891,-0.262017358841779,
-2.58941709788185));
#7714=CARTESIAN_POINT('Ctrl Pts',(-26.8857631894022,-0.277848484290429,
-2.58714012203648));
#7715=CARTESIAN_POINT('Ctrl Pts',(-26.8713173449163,-0.324894779397646,
-2.5797790328415));
#7716=CARTESIAN_POINT('Ctrl Pts',(-26.8601819442124,-0.355668892391165,
-2.57416342317005));
#7717=CARTESIAN_POINT('Ctrl Pts',(-26.8412486366545,-0.400939993511204,
-2.56479183005489));
#7718=CARTESIAN_POINT('Ctrl Pts',(-26.8345590268073,-0.415893141702949,
-2.56150689497223));
#7719=CARTESIAN_POINT('Ctrl Pts',(-26.823967020712,-0.438089012396736,-2.55635832654132));
#7720=CARTESIAN_POINT('Ctrl Pts',(-26.8203396689083,-0.445455430851165,
-2.55460350724556));
#7721=CARTESIAN_POINT('Ctrl Pts',(-26.8128985600938,-0.460108665512354,
-2.55102277071131));
#7722=CARTESIAN_POINT('Ctrl Pts',(-26.8090795604559,-0.467404628169114,
-2.54919438667112));
#7723=CARTESIAN_POINT('Ctrl Pts',(-26.797394241101,-0.489073962305609,-2.54363152212406));
#7724=CARTESIAN_POINT('Ctrl Pts',(-26.789289060049,-0.503254782620716,-2.53981402566019));
#7725=CARTESIAN_POINT('Ctrl Pts',(-26.7724543674525,-0.531113894213054,
-2.53198595664959));
#7726=CARTESIAN_POINT('Ctrl Pts',(-26.7637261115164,-0.54479019657989,-2.52797594056182));
#7727=CARTESIAN_POINT('Ctrl Pts',(-26.7366204601151,-0.585077837829173,
-2.51569932133657));
#7728=CARTESIAN_POINT('Ctrl Pts',(-26.7173245039422,-0.610949544590535,
-2.50718576295211));
#7729=CARTESIAN_POINT('Ctrl Pts',(-26.6865409768543,-0.648314158915969,
-2.49408419229669));
#7730=CARTESIAN_POINT('Ctrl Pts',(-26.6759726166714,-0.660528085389519,
-2.48966171422195));
#7731=CARTESIAN_POINT('Ctrl Pts',(-26.6542132239272,-0.684474388015635,
-2.48073390605899));
#7732=CARTESIAN_POINT('Ctrl Pts',(-26.6430264626965,-0.696202382055651,
-2.4762302346818));
#7733=CARTESIAN_POINT('Ctrl Pts',(-26.6257563658622,-0.713443816566624,
-2.46942885891314));
#7734=CARTESIAN_POINT('Ctrl Pts',(-26.6199203558455,-0.719129338058233,
-2.46715519418602));
#7735=CARTESIAN_POINT('Ctrl Pts',(-26.6081482145809,-0.730321546007048,
-2.46262131897029));
#7736=CARTESIAN_POINT('Ctrl Pts',(-26.602201292566,-0.735839132509799,-2.46035683871519));
#7737=CARTESIAN_POINT('Ctrl Pts',(-26.5841980514885,-0.752140229430926,
-2.45358395979734));
#7738=CARTESIAN_POINT('Ctrl Pts',(-26.5719627057113,-0.76268889323127,-2.44908952535157));
#7739=CARTESIAN_POINT('Ctrl Pts',(-26.5345850153881,-0.793372503429244,
-2.43572354204093));
#7740=CARTESIAN_POINT('Ctrl Pts',(-26.5087533968938,-0.812566724291243,
-2.42696101356095));
#7741=CARTESIAN_POINT('Ctrl Pts',(-26.4686207796459,-0.839482273044303,
-2.41422655155215));
#7742=CARTESIAN_POINT('Ctrl Pts',(-26.4550114406092,-0.848141391767849,
-2.4100497583254));
#7743=CARTESIAN_POINT('Ctrl Pts',(-26.4273190367366,-0.864830292639691,
-2.40186446327311));
#7744=CARTESIAN_POINT('Ctrl Pts',(-26.4132360104195,-0.872860114977224,
-2.39785591495116));
#7745=CARTESIAN_POINT('Ctrl Pts',(-26.384582055835,-0.888281159414981,-2.39004076104538));
#7746=CARTESIAN_POINT('Ctrl Pts',(-26.3700168965852,-0.895669478070542,
-2.38623564655444));
#7747=CARTESIAN_POINT('Ctrl Pts',(-26.3477718580352,-0.906270310920242,
-2.38070172959633));
#7748=CARTESIAN_POINT('Ctrl Pts',(-26.3402920246762,-0.909722137727464,
-2.3788867625548));
#7749=CARTESIAN_POINT('Ctrl Pts',(-26.3252941333419,-0.9164202866514,-2.37534201103856));
#7750=CARTESIAN_POINT('Ctrl Pts',(-26.3177603512233,-0.919674724840889,
-2.37360807070524));
#7751=CARTESIAN_POINT('Ctrl Pts',(-26.2799597723219,-0.935450414400054,
-2.36515131650746));
#7752=CARTESIAN_POINT('Ctrl Pts',(-26.2492303116149,-0.946538086235367,
-2.35904259359383));
#7753=CARTESIAN_POINT('Ctrl Pts',(-26.1868085832625,-0.965668578368493,
-2.34833591063874));
#7754=CARTESIAN_POINT('Ctrl Pts',(-26.1551124003162,-0.973715224519596,
-2.34373600934578));
#7755=CARTESIAN_POINT('Ctrl Pts',(-26.1068141625445,-0.983466877886542,
-2.33810786542035));
#7756=CARTESIAN_POINT('Ctrl Pts',(-26.0905889199931,-0.986330406808508,
-2.33644376922427));
#7757=CARTESIAN_POINT('Ctrl Pts',(-26.0578798138569,-0.991267004789945,
-2.33356356824837));
#7758=CARTESIAN_POINT('Ctrl Pts',(-26.0413987784432,-0.993339559141272,
-2.33234779729885));
#7759=CARTESIAN_POINT('Ctrl Pts',(-26.0164682576784,-0.995840021233339,
-2.33087747927257));
#7760=CARTESIAN_POINT('Ctrl Pts',(-26.0081136505026,-0.996572064821672,
-2.33044626591382));
#7761=CARTESIAN_POINT('Ctrl Pts',(-25.9914405419907,-0.997822188899729,
-2.3297091449783));
#7762=CARTESIAN_POINT('Ctrl Pts',(-25.983108979154,-0.998341962394754,-2.32940224532968));
#7763=CARTESIAN_POINT('Ctrl Pts',(-25.9581619401288,-0.999585267481811,
-2.32866771122069));
#7764=CARTESIAN_POINT('Ctrl Pts',(-25.9415535530913,-0.999997281825196,
-2.32842370354953));
#7765=CARTESIAN_POINT('Ctrl Pts',(-25.8918801633427,-0.999995995609914,
-2.32842452644233));
#7766=CARTESIAN_POINT('Ctrl Pts',(-25.8588977400795,-0.998354960350017,
-2.32939847806693));
#7767=CARTESIAN_POINT('Ctrl Pts',(-25.809655632564,-0.993459342757443,-2.33227744379061));
#7768=CARTESIAN_POINT('Ctrl Pts',(-25.7932782734797,-0.991421278478376,
-2.33347323218692));
#7769=CARTESIAN_POINT('Ctrl Pts',(-25.7605969584102,-0.986528474355795,
-2.33632851316856));
#7770=CARTESIAN_POINT('Ctrl Pts',(-25.7442875327586,-0.983672349909108,
-2.33798881805762));
#7771=CARTESIAN_POINT('Ctrl Pts',(-25.7198951962202,-0.97877216559872,-2.34081761913493));
#7772=CARTESIAN_POINT('Ctrl Pts',(-25.7117696482312,-0.977034217384623,
-2.34181798163729));
#7773=CARTESIAN_POINT('Ctrl Pts',(-25.6955367491711,-0.973349801421778,
-2.34393091101302));
#7774=CARTESIAN_POINT('Ctrl Pts',(-25.6874344702097,-0.971403984435828,
-2.34504307866984));
#7775=CARTESIAN_POINT('Ctrl Pts',(-25.6632988267017,-0.965288201987582,
-2.34852442457186));
#7776=CARTESIAN_POINT('Ctrl Pts',(-25.6473898327442,-0.960831588438292,
-2.35104334024925));
#7777=CARTESIAN_POINT('Ctrl Pts',(-25.6159256353873,-0.951177087518217,
-2.35644596476354));
#7778=CARTESIAN_POINT('Ctrl Pts',(-25.6003698930602,-0.945979355455216,
-2.35932958924631));
#7779=CARTESIAN_POINT('Ctrl Pts',(-25.5696016033233,-0.934854907919286,
-2.36543090574196));
#7780=CARTESIAN_POINT('Ctrl Pts',(-25.5543890761051,-0.928928152287276,
-2.36864862443056));
#7781=CARTESIAN_POINT('Ctrl Pts',(-25.5092559713361,-0.910063051819414,
-2.37875853937476));
#7782=CARTESIAN_POINT('Ctrl Pts',(-25.4798371327009,-0.896039907812134,
-2.3861084711256));
#7783=CARTESIAN_POINT('Ctrl Pts',(-25.4438916664408,-0.876696452792308,
-2.39591178467008));
#7784=CARTESIAN_POINT('Ctrl Pts',(-25.4367422081294,-0.872734553740174,
-2.39790417870508));
#7785=CARTESIAN_POINT('Ctrl Pts',(-25.4225301197978,-0.864630295332379,
-2.40194577660712));
#7786=CARTESIAN_POINT('Ctrl Pts',(-25.415458892085,-0.860482058534017,-2.40399774819589));
#7787=CARTESIAN_POINT('Ctrl Pts',(-25.3944665440157,-0.84781813222127,-2.41020698379142));
#7788=CARTESIAN_POINT('Ctrl Pts',(-25.3807469194853,-0.839074603637404,
-2.41442221810217));
#7789=CARTESIAN_POINT('Ctrl Pts',(-25.3538269146123,-0.820986612312255,
-2.42297440207295));
#7790=CARTESIAN_POINT('Ctrl Pts',(-25.3406288513095,-0.811643743807895,
-2.42731061510823));
#7791=CARTESIAN_POINT('Ctrl Pts',(-25.3147440120878,-0.792365407430333,
-2.43607078110781));
#7792=CARTESIAN_POINT('Ctrl Pts',(-25.302057253131,-0.782429927595734,-2.44049476170448));
#7793=CARTESIAN_POINT('Ctrl Pts',(-25.2771870451046,-0.761966360498884,
-2.44939937123357));
#7794=CARTESIAN_POINT('Ctrl Pts',(-25.2650036031527,-0.751438272731148,
-2.45388002625663));
#7795=CARTESIAN_POINT('Ctrl Pts',(-25.2411363975391,-0.729784484637608,
-2.4628677672137));
#7796=CARTESIAN_POINT('Ctrl Pts',(-25.2294526316117,-0.718658795136046,
-2.46737487908639));
#7797=CARTESIAN_POINT('Ctrl Pts',(-25.2065854499521,-0.695799709481919,
-2.47638573024674));
#7798=CARTESIAN_POINT('Ctrl Pts',(-25.1954025574532,-0.684066558646475,
-2.48088932142673));
#7799=CARTESIAN_POINT('Ctrl Pts',(-25.1790057014816,-0.665998774177092,
-2.48762031005077));
#7800=CARTESIAN_POINT('Ctrl Pts',(-25.1735972102192,-0.659890699564593,
-2.48986242816921));
#7801=CARTESIAN_POINT('Ctrl Pts',(-25.162950610077,-0.647566600651535,-2.49431653723256));
#7802=CARTESIAN_POINT('Ctrl Pts',(-25.157711714779,-0.641350879252792,-2.49652867473458));
#7803=CARTESIAN_POINT('Ctrl Pts',(-25.1319370754269,-0.609998354557005,
-2.50750690290623));
#7804=CARTESIAN_POINT('Ctrl Pts',(-25.1126444312025,-0.584052119288394,
-2.51602690308558));
#7805=CARTESIAN_POINT('Ctrl Pts',(-25.0766572872409,-0.530427486923969,
-2.53233703039074));
#7806=CARTESIAN_POINT('Ctrl Pts',(-25.059961236299,-0.502749651254318,-2.5401282199127));
#7807=CARTESIAN_POINT('Ctrl Pts',(-25.0368800991623,-0.459893940418667,
-2.5511186769858));
#7808=CARTESIAN_POINT('Ctrl Pts',(-25.0295141239499,-0.445385200926373,
-2.55466616380488));
#7809=CARTESIAN_POINT('Ctrl Pts',(-25.0154489582634,-0.415908528063236,
-2.56150305960081));
#7810=CARTESIAN_POINT('Ctrl Pts',(-25.0087494145486,-0.40093905147491,-2.56479267814123));
#7811=CARTESIAN_POINT('Ctrl Pts',(-24.999213902548,-0.378133256488478,-2.56951273362109));
#7812=CARTESIAN_POINT('Ctrl Pts',(-24.9961168386391,-0.370460488165637,
-2.57105248627293));
#7813=CARTESIAN_POINT('Ctrl Pts',(-24.9901160989215,-0.355044978918729,
-2.57404734396979));
#7814=CARTESIAN_POINT('Ctrl Pts',(-24.9872176813169,-0.34731693891287,-2.57549979202268));
#7815=CARTESIAN_POINT('Ctrl Pts',(-24.978825003649,-0.324068265856262,-2.57972038676599));
#7816=CARTESIAN_POINT('Ctrl Pts',(-24.9736233181388,-0.308461431450075,
-2.5823566152535));
#7817=CARTESIAN_POINT('Ctrl Pts',(-24.9640114746886,-0.277068877280409,
-2.58725544515497));
#7818=CARTESIAN_POINT('Ctrl Pts',(-24.9595988320509,-0.261277274869767,
-2.58951929498313));
#7819=CARTESIAN_POINT('Ctrl Pts',(-24.9515558748387,-0.229503410355288,
-2.59366439634912));
#7820=CARTESIAN_POINT('Ctrl Pts',(-24.9479255650923,-0.213521148150432,
-2.59554565951958));
#7821=CARTESIAN_POINT('Ctrl Pts',(-24.9414489760593,-0.181364697617433,
-2.59891367071842));
#7822=CARTESIAN_POINT('Ctrl Pts',(-24.9386026892397,-0.165190511764201,
-2.60040043074177));
#7823=CARTESIAN_POINT('Ctrl Pts',(-24.9337017706774,-0.132647674346382,
-2.60296683712999));
#7824=CARTESIAN_POINT('Ctrl Pts',(-24.9316471184334,-0.116279028004551,
-2.60404649646001));
#7825=CARTESIAN_POINT('Ctrl Pts',(-24.9283432634801,-0.0833433888462472,
-2.60578520034254));
#7826=CARTESIAN_POINT('Ctrl Pts',(-24.9270943388138,-0.0667755622802253,
-2.60644409327794));
#7827=CARTESIAN_POINT('Ctrl Pts',(-24.9258394406481,-0.0417735825487939,
-2.60710648445229));
#7828=CARTESIAN_POINT('Ctrl Pts',(-24.9255244961035,-0.0334015655269927,
-2.6072728288538));
#7829=CARTESIAN_POINT('Ctrl Pts',(-24.9251056202904,-0.0166741410701568,
-2.60749409590418));
#7830=CARTESIAN_POINT('Ctrl Pts',(-24.9250013822027,-0.00832706674008044,
-2.60754917994845));
#7831=CARTESIAN_POINT('Ctrl Pts',(-24.9250015605239,9.19874578470569E-16,
-2.60754908509523));
#7832=CARTESIAN_POINT('Origin',(-28.425,5.02797759097482E-32,0.));
#7833=CARTESIAN_POINT('',(-28.425,-3.,1.00000000000001));
#7834=CARTESIAN_POINT('Origin',(-28.425,-3.,1.00000000000001));
#7835=CARTESIAN_POINT('',(-21.125,-3.,0.999999999999995));
#7836=CARTESIAN_POINT('Origin',(-21.125,-3.,-1.00000000000001));
#7837=CARTESIAN_POINT('',(-21.125,-3.,-1.00000000000001));
#7838=CARTESIAN_POINT('Origin',(-28.425,-3.,-1.00000000000001));
#7839=CARTESIAN_POINT('',(-28.425,-3.,-1.00000000000001));
#7840=CARTESIAN_POINT('Origin',(-28.425,5.02797759097482E-32,0.));
#10535=UNCERTAINTY_MEASURE_WITH_UNIT(LENGTH_MEASURE(0.01),#10552,
'DISTANCE_ACCURACY_VALUE',
'Maximum model space distance between geometric entities at asserted c
onnectivities');
#10540=UNCERTAINTY_MEASURE_WITH_UNIT(LENGTH_MEASURE(0.01),#10552,
'DISTANCE_ACCURACY_VALUE',
'Maximum model space distance between geometric entities at asserted c
onnectivities');
#10546=(
GEOMETRIC_REPRESENTATION_CONTEXT(3)
GLOBAL_UNCERTAINTY_ASSIGNED_CONTEXT((#10535))
GLOBAL_UNIT_ASSIGNED_CONTEXT((#10552,#10554,#10555))
REPRESENTATION_CONTEXT('','3D')
);
#10551=(
GEOMETRIC_REPRESENTATION_CONTEXT(3)
GLOBAL_UNCERTAINTY_ASSIGNED_CONTEXT((#10540))
GLOBAL_UNIT_ASSIGNED_CONTEXT((#10552,#10554,#10555))
REPRESENTATION_CONTEXT('','3D')
);
#10552=(
LENGTH_UNIT()
NAMED_UNIT(*)
SI_UNIT(.MILLI.,.METRE.)
);
#10554=(
NAMED_UNIT(*)
PLANE_ANGLE_UNIT()
SI_UNIT($,.RADIAN.)
);
#10555=(
NAMED_UNIT(*)
SI_UNIT($,.STERADIAN.)
SOLID_ANGLE_UNIT()
);
#10561=SHAPE_DEFINITION_REPRESENTATION(#10571,#10590);
#10571=PRODUCT_DEFINITION_SHAPE('',$,#10601);
#10590=SHAPE_REPRESENTATION('',(#3651),#10546);
#10595=PRODUCT_DEFINITION_CONTEXT('part definition',#10627,'design');
#10601=PRODUCT_DEFINITION('Plunger','Plunger',#10611,#10595);
#10611=PRODUCT_DEFINITION_FORMATION('',$,#10634);
#10627=APPLICATION_CONTEXT(
'Core Data for Automotive Mechanical Design Process');
#10628=PRODUCT_CONTEXT('part definition',#10627,'mechanical');
#10634=PRODUCT('Plunger','Plunger',$,(#10628));
#10643=PRESENTATION_STYLE_ASSIGNMENT((#10650));
#10650=SURFACE_STYLE_USAGE(.BOTH.,#10657);
#10657=SURFACE_SIDE_STYLE('',(#10664));
#10664=SURFACE_STYLE_FILL_AREA(#10671);
#10671=FILL_AREA_STYLE('Opaque(61,176,222)',(#10678));
#10678=FILL_AREA_STYLE_COLOUR('Opaque(61,176,222)',#10685);
#10685=COLOUR_RGB('Opaque(61,176,222)',0.23921568627451,0.690196078431373,
0.870588235294118);
ENDSEC;
END-ISO-10303-21;
